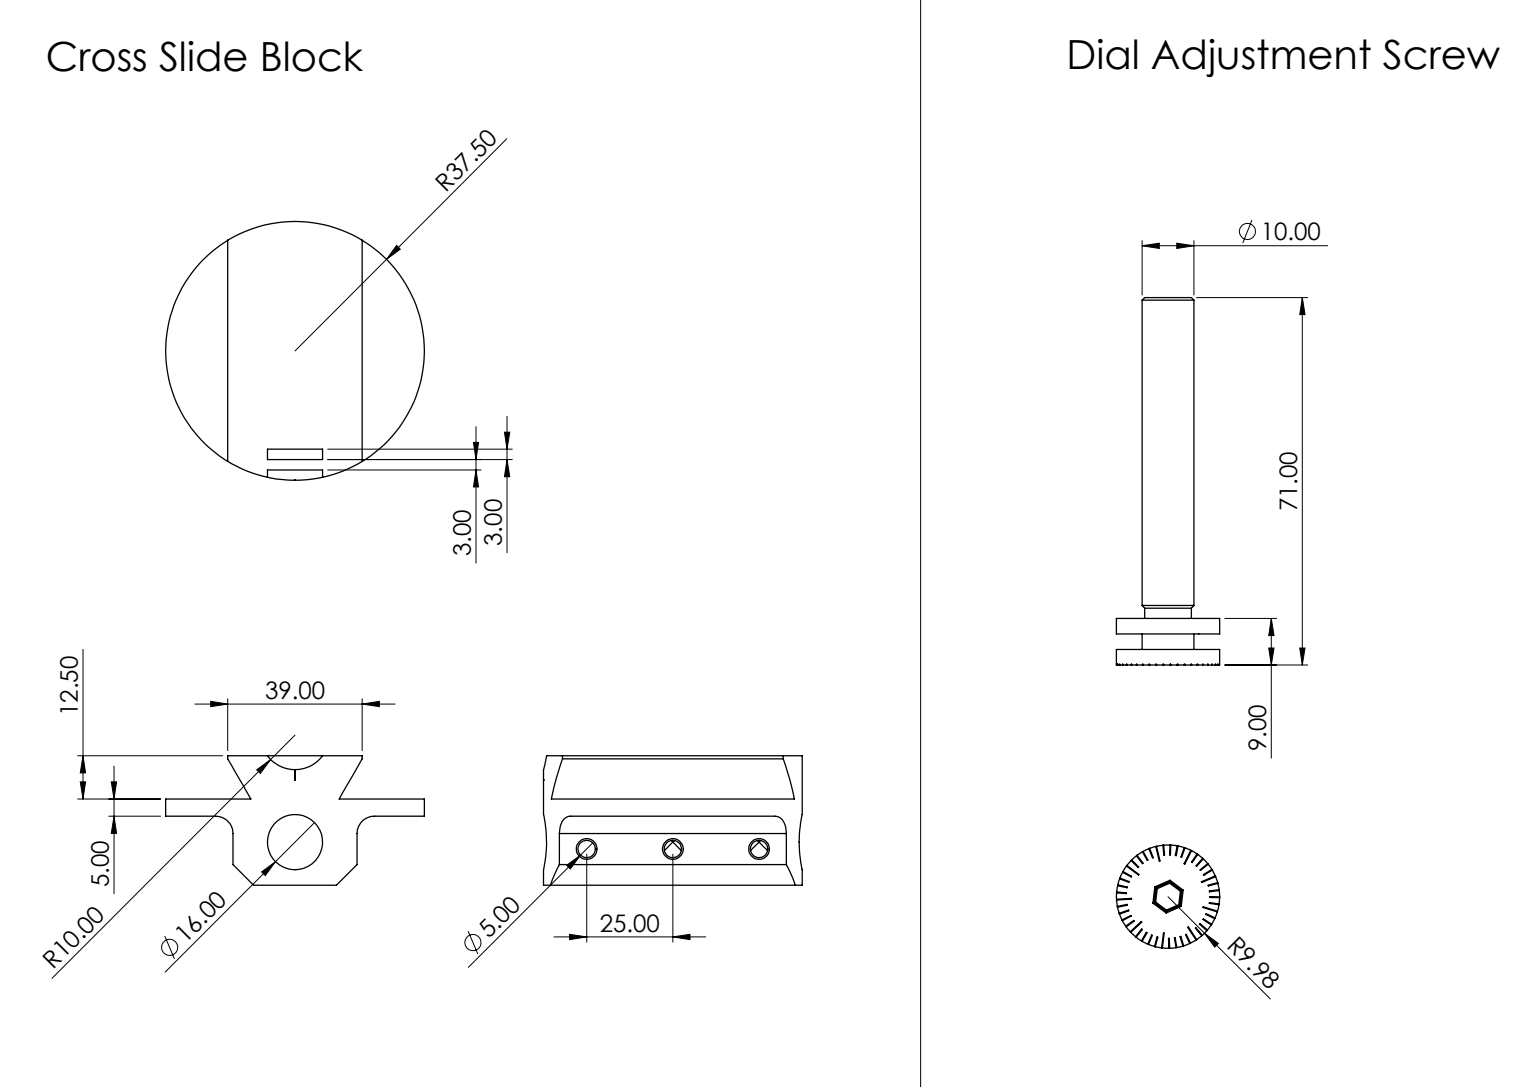
ISO-10303-21;
HEADER;
FILE_DESCRIPTION (('STEP AP214'),
    '1' );
FILE_NAME ('Cross Slide Block.step',
    '2026-10-09T18:50:44',
    ( '' ),
    ( '' ),
    'SwSTEP 2.0',
    'SolidWorks 2026',
    '' );
FILE_SCHEMA (( 'AUTOMOTIVE_DESIGN' ));
ENDSEC;

DATA;
#2=ADVANCED_FACE ( 'NONE', ( #7489 ), #472, .F. ) ;
#3=FACE_OUTER_BOUND ( 'NONE', #3774, .T. ) ;
#5=( BOUNDED_CURVE ( )  B_SPLINE_CURVE ( 3, ( #1335, #9589, #4703, #9365 ),
 .UNSPECIFIED., .F., .F. ) 
 B_SPLINE_CURVE_WITH_KNOTS ( ( 4, 4 ),
 ( 1.628044839356179940, 3.141592653589793116 ),
 .UNSPECIFIED. ) 
 CURVE ( )  GEOMETRIC_REPRESENTATION_ITEM ( )  RATIONAL_B_SPLINE_CURVE ( ( 1.000000000000000000, 0.8180365063541270576, 0.8180365063541270576, 1.000000000000000000 ) ) 
 REPRESENTATION_ITEM ( '' )  );
#9=CARTESIAN_POINT ( 'NONE',  ( -36.90121799483238618, -37.26927769664154511, 50.29562344872909563 ) ) ;
#16=EDGE_CURVE ( 'NONE', #234, #9567, #717, .T. ) ;
#23=CARTESIAN_POINT ( 'NONE',  ( 2.500300139188999182, -51.00737899243799944, -13.39525803434800011 ) ) ;
#28=CARTESIAN_POINT ( 'NONE',  ( -21.52984724227062685, -49.79067269186487721, -17.51158402248789869 ) ) ;
#37=CARTESIAN_POINT ( 'NONE',  ( -15.57469986081333424, -23.50709773848279482, 57.00223526477140013 ) ) ;
#38=EDGE_CURVE ( 'NONE', #4941, #11428, #1756, .T. ) ;
#42=CARTESIAN_POINT ( 'NONE',  ( -7.506852801849951184, -44.86566843535796778, 21.38792573514972872 ) ) ;
#48=EDGE_LOOP ( 'NONE', ( #7800, #11011, #11564, #11938, #6650, #9579, #4015 ) ) ;
#51=FACE_BOUND ( 'NONE', #14476, .T. ) ;
#53=CARTESIAN_POINT ( 'NONE',  ( -10.22150846799388191, -38.48997916076172743, -17.62493476913342150 ) ) ;
#64=VECTOR ( 'NONE', #10695, 1000.000000000000000 ) ;
#74=CARTESIAN_POINT ( 'NONE',  ( -5.499699860811000818, -46.50737899243799944, 22.50231026484399877 ) ) ;
#82=FACE_OUTER_BOUND ( 'NONE', #1702, .T. ) ;
#95=ORIENTED_EDGE ( 'NONE', *, *, #10374, .T. ) ;
#99=( BOUNDED_CURVE ( )  B_SPLINE_CURVE ( 3, ( #13212, #2486, #10670, #275 ),
 .UNSPECIFIED., .F., .T. ) 
 B_SPLINE_CURVE_WITH_KNOTS ( ( 4, 4 ),
 ( 4.712388980384689674, 6.283185307179586232 ),
 .UNSPECIFIED. ) 
 CURVE ( )  GEOMETRIC_REPRESENTATION_ITEM ( )  RATIONAL_B_SPLINE_CURVE ( ( 1.000000000000000000, 0.8047378541243649375, 0.8047378541243649375, 1.000000000000000000 ) ) 
 REPRESENTATION_ITEM ( '' )  );
#104=AXIS2_PLACEMENT_3D ( 'NONE', #5495, #8007, #12779 ) ;
#108=ORIENTED_EDGE ( 'NONE', *, *, #1414, .F. ) ;
#111=AXIS2_PLACEMENT_3D ( 'NONE', #10208, #14881, #11508 ) ;
#112=ORIENTED_EDGE ( 'NONE', *, *, #3083, .T. ) ;
#116=CARTESIAN_POINT ( 'NONE',  ( 4.650967236384746073, -37.88568168827513460, 51.12989147907354948 ) ) ;
#125=CARTESIAN_POINT ( 'NONE',  ( -7.500433020662222283, -49.00523987278725713, -5.609464624471996785 ) ) ;
#126=LINE ( 'NONE', #11658, #7291 ) ;
#128=DIRECTION ( 'NONE',  ( 0.000000000000000000, 0.000000000000000000, -1.000000000000000000 ) ) ;
#151=CARTESIAN_POINT ( 'NONE',  ( 2.500300139188999182, -51.00737899243799944, -13.39525803434800011 ) ) ;
#153=CARTESIAN_POINT ( 'NONE',  ( -28.28282149594069850, -32.00737899243799944, -17.99768973515599768 ) ) ;
#162=LINE ( 'NONE', #9710, #2630 ) ;
#163=CARTESIAN_POINT ( 'NONE',  ( -37.26807582031575805, -37.15669500878452425, 50.03818627108570638 ) ) ;
#172=ORIENTED_EDGE ( 'NONE', *, *, #3900, .F. ) ;
#174=CARTESIAN_POINT ( 'NONE',  ( -15.49969986081099904, -44.50737899243799944, -109.5506571639849938 ) ) ;
#177=EDGE_CURVE ( 'NONE', #13055, #12587, #8525, .T. ) ;
#182=CARTESIAN_POINT ( 'NONE',  ( 4.224496369445544630, -38.22985747236960918, -12.39136299437819488 ) ) ;
#187=CARTESIAN_POINT ( 'NONE',  ( 2.883830742001312508, -40.08477038827061989, 52.18712618527332125 ) ) ;
#189=CIRCLE ( 'NONE', #12147, 2.499999999999999556 ) ;
#199=EDGE_LOOP ( 'NONE', ( #11824, #6464, #11368, #3598 ) ) ;
#202=CARTESIAN_POINT ( 'NONE',  ( -7.499699860810999041, -19.50737899243799589, 51.00231026484400587 ) ) ;
#206=CARTESIAN_POINT ( 'NONE',  ( -16.55248250669792753, -52.45523696625489407, 56.99108552064786437 ) ) ;
#208=( NAMED_UNIT ( * ) SI_UNIT ( $, .STERADIAN. ) SOLID_ANGLE_UNIT ( ) );
#213=CARTESIAN_POINT ( 'NONE',  ( -15.49969986081099016, -52.50737899243799944, 27.50231026484399521 ) ) ;
#214=EDGE_CURVE ( 'NONE', #2810, #1679, #14130, .T. ) ;
#226=CARTESIAN_POINT ( 'NONE',  ( -15.49969986081098838, -17.75737899243799944, 48.00231026484399877 ) ) ;
#229=CARTESIAN_POINT ( 'NONE',  ( -7.753733168396170328, -46.50737899243799944, 47.00231026484399877 ) ) ;
#231=AXIS2_PLACEMENT_3D ( 'NONE', #5849, #3193, #3340 ) ;
#232=PLANE ( 'NONE',  #13853 ) ;
#234=VERTEX_POINT ( 'NONE', #10472 ) ;
#237=CARTESIAN_POINT ( 'NONE',  ( -15.49969986081099727, -52.50737899243799944, 2.502310264843994769 ) ) ;
#240=VECTOR ( 'NONE', #12413, 1000.000000000000000 ) ;
#243=ORIENTED_EDGE ( 'NONE', *, *, #13545, .T. ) ;
#244=ORIENTED_EDGE ( 'NONE', *, *, #12022, .T. ) ;
#253=CIRCLE ( 'NONE', #14173, 37.50000000000000000 ) ;
#260=ORIENTED_EDGE ( 'NONE', *, *, #6343, .T. ) ;
#261=CARTESIAN_POINT ( 'NONE',  ( 5.515696375138871232, -37.41693849659856141, 50.56059116161328859 ) ) ;
#272=CARTESIAN_POINT ( 'NONE',  ( -7.749729581313432369, -48.02091033734640035, -3.487279356396127739 ) ) ;
#273=CARTESIAN_POINT ( 'NONE',  ( -34.99969986081099904, -19.50737899243800300, 51.53354502093799994 ) ) ;
#275=CARTESIAN_POINT ( 'NONE',  ( -15.49969986081099727, -36.50737899243799944, 2.502310264843996546 ) ) ;
#279=CARTESIAN_POINT ( 'NONE',  ( -5.499699860811003482, -46.50737899243799944, 44.50231026484399877 ) ) ;
#281=CARTESIAN_POINT ( 'NONE',  ( -14.45170227088251202, -36.55910949265851428, -17.98655532003696678 ) ) ;
#283=EDGE_CURVE ( 'NONE', #10750, #11940, #6056, .T. ) ;
#285=DIRECTION ( 'NONE',  ( 0.000000000000000000, 0.000000000000000000, -1.000000000000000000 ) ) ;
#297=ORIENTED_EDGE ( 'NONE', *, *, #1602, .F. ) ;
#299=ORIENTED_EDGE ( 'NONE', *, *, #12335, .F. ) ;
#314=ADVANCED_FACE ( 'NONE', ( #7004, #5865, #10542, #6834 ), #10286, .F. ) ;
#318=ORIENTED_EDGE ( 'NONE', *, *, #7751, .T. ) ;
#338=CARTESIAN_POINT ( 'NONE',  ( -15.49969986081099904, -57.00737899243801365, 57.00231026484399166 ) ) ;
#344=ORIENTED_EDGE ( 'NONE', *, *, #5377, .F. ) ;
#363=CARTESIAN_POINT ( 'NONE',  ( -19.50440554761897261, -37.57692853466172522, 56.78858631758297548 ) ) ;
#376=DIRECTION ( 'NONE',  ( 0.000000000000000000, 0.000000000000000000, 1.000000000000000000 ) ) ;
#379=PLANE ( 'NONE',  #13903 ) ;
#384=DIRECTION ( 'NONE',  ( 0.000000000000000000, -1.000000000000000000, -1.224646799147350002E-16 ) ) ;
#386=CARTESIAN_POINT ( 'NONE',  ( -7.813858722443232097, -47.64803766822201680, 17.27706589258430014 ) ) ;
#387=LINE ( 'NONE', #9553, #4308 ) ;
#390=CARTESIAN_POINT ( 'NONE',  ( -7.921791253741313987, -47.08507903579843656, -17.22412991407007254 ) ) ;
#393=EDGE_CURVE ( 'NONE', #2126, #6515, #10210, .T. ) ;
#397=CARTESIAN_POINT ( 'NONE',  ( -33.53898029810832782, -41.37673382704548430, -13.37373704449904999 ) ) ;
#399=ORIENTED_EDGE ( 'NONE', *, *, #9618, .F. ) ;
#410=SHAPE_REPRESENTATION ( 'Cross Slide Block', ( #6789 ), #14627 ) ;
#411=DIRECTION ( 'NONE',  ( 0.000000000000000000, -1.000000000000000000, -1.224646799147350002E-16 ) ) ;
#424=CARTESIAN_POINT ( 'NONE',  ( -7.499751500627866996, -49.00722532478560822, -5.529656340655102476 ) ) ;
#427=CARTESIAN_POINT ( 'NONE',  ( 2.500300139188998738, -46.50737899243799944, 22.00231026484399877 ) ) ;
#435=ADVANCED_FACE ( 'NONE', ( #3259 ), #11815, .F. ) ;
#437=CARTESIAN_POINT ( 'NONE',  ( -9.503465417293824657, -21.51087798686868169, 56.51956357228300476 ) ) ;
#455=AXIS2_PLACEMENT_3D ( 'NONE', #5725, #6934, #3584 ) ;
#458=ADVANCED_FACE ( 'NONE', ( #3557 ), #9287, .T. ) ;
#459=CARTESIAN_POINT ( 'NONE',  ( -7.879287384819388507, -47.08648443922106708, 17.06717620651851064 ) ) ;
#461=DIRECTION ( 'NONE',  ( -1.000000000000000000, 1.291538348938060198E-32, -1.054621095516909827E-16 ) ) ;
#463=DIRECTION ( 'NONE',  ( 0.000000000000000000, 0.000000000000000000, 1.000000000000000000 ) ) ;
#468=CARTESIAN_POINT ( 'NONE',  ( -37.32932784798677517, -37.10979894228395182, -10.99641364132881094 ) ) ;
#472=CYLINDRICAL_SURFACE ( 'NONE', #13911, 10.00000000000000000 ) ;
#477=CYLINDRICAL_SURFACE ( 'NONE', #7239, 2.500000000000002220 ) ;
#483=CARTESIAN_POINT ( 'NONE',  ( -7.506367692296740834, -44.17806943360024974, 45.42009090809814609 ) ) ;
#486=CARTESIAN_POINT ( 'NONE',  ( -1.425463962227843995, -54.93314309385483796, 54.32987364559348009 ) ) ;
#496=( BOUNDED_CURVE ( )  B_SPLINE_CURVE ( 3, ( #7778, #12464, #6703, #906 ),
 .UNSPECIFIED., .F., .F. ) 
 B_SPLINE_CURVE_WITH_KNOTS ( ( 4, 4 ),
 ( 1.570796326794895004, 3.141592653589793116 ),
 .UNSPECIFIED. ) 
 CURVE ( )  GEOMETRIC_REPRESENTATION_ITEM ( )  RATIONAL_B_SPLINE_CURVE ( ( 1.000000000000000000, 0.8047378541243646044, 0.8047378541243646044, 1.000000000000000000 ) ) 
 REPRESENTATION_ITEM ( '' )  );
#504=CARTESIAN_POINT ( 'NONE',  ( -21.84916367058906772, -49.38105347906694931, 56.46124168193669135 ) ) ;
#515=EDGE_CURVE ( 'NONE', #12112, #5496, #126, .T. ) ;
#518=ORIENTED_EDGE ( 'NONE', *, *, #13012, .T. ) ;
#521=CARTESIAN_POINT ( 'NONE',  ( -7.838590061662593200, -46.81644859005926662, 21.98773677246508740 ) ) ;
#542=PRODUCT_DEFINITION_SHAPE ( 'NONE', 'NONE',  #10680 ) ;
#546=CARTESIAN_POINT ( 'NONE',  ( -5.499699860811000818, -46.50737899243799944, 22.50231026484399877 ) ) ;
#548=FACE_OUTER_BOUND ( 'NONE', #4580, .T. ) ;
#569=VERTEX_POINT ( 'NONE', #273 ) ;
#570=CARTESIAN_POINT ( 'NONE',  ( -15.49969986081099371, -26.50737899243800300, 56.85231026484400019 ) ) ;
#573=CARTESIAN_POINT ( 'NONE',  ( -5.499699860810998153, -46.50737899243799944, -2.497689735156003010 ) ) ;
#576=CARTESIAN_POINT ( 'NONE',  ( -18.33272512729327985, -51.99348705970457729, 56.89592189784066534 ) ) ;
#577=ORIENTED_EDGE ( 'NONE', *, *, #2278, .F. ) ;
#578=CARTESIAN_POINT ( 'NONE',  ( -14.97634376076197427, -36.52016005446672864, 56.99957717010889269 ) ) ;
#589=DIRECTION ( 'NONE',  ( -3.839882694219489529E-17, 1.000000000000000000, 0.000000000000000000 ) ) ;
#603=CARTESIAN_POINT ( 'NONE',  ( 2.500300139188996962, -46.50737899243799944, 41.50231026484399166 ) ) ;
#608=VECTOR ( 'NONE', #7086, 1000.000000000000000 ) ;
#610=CARTESIAN_POINT ( 'NONE',  ( -35.12686845230359722, -38.31628777931871355, -12.45116519455210202 ) ) ;
#623=CARTESIAN_POINT ( 'NONE',  ( -7.500891366873055688, -44.35589769198639942, 43.22203397690024218 ) ) ;
#624=ORIENTED_EDGE ( 'NONE', *, *, #10374, .F. ) ;
#632=DIRECTION ( 'NONE',  ( 0.000000000000000000, 0.000000000000000000, -1.000000000000000000 ) ) ;
#648=EDGE_LOOP ( 'NONE', ( #4869, #13209, #1415, #10166, #10438, #12905, #14791, #3642, #7670 ) ) ;
#649=CARTESIAN_POINT ( 'NONE',  ( -13.41733751443047318, -36.76536173621014569, 56.94798727393903448 ) ) ;
#654=AXIS2_PLACEMENT_3D ( 'NONE', #10348, #4542, #5827 ) ;
#658=FACE_OUTER_BOUND ( 'NONE', #3242, .T. ) ;
#661=ORIENTED_EDGE ( 'NONE', *, *, #914, .T. ) ;
#677=CARTESIAN_POINT ( 'NONE',  ( -7.557949836157023427, -45.46309933671603432, -3.215436967628607867 ) ) ;
#681=FACE_OUTER_BOUND ( 'NONE', #12815, .T. ) ;
#684=EDGE_CURVE ( 'NONE', #5678, #1019, #2058, .T. ) ;
#687=CARTESIAN_POINT ( 'NONE',  ( -11.90127153857800302, -52.50737899243802786, 27.50231026484402719 ) ) ;
#697=CARTESIAN_POINT ( 'NONE',  ( -7.499699860810999041, -44.50737899243799944, 43.00231026484400587 ) ) ;
#698=ORIENTED_EDGE ( 'NONE', *, *, #7230, .T. ) ;
#702=CARTESIAN_POINT ( 'NONE',  ( -7.661871090851159138, -46.13481490855701139, -7.997691309909533253 ) ) ;
#716=CARTESIAN_POINT ( 'NONE',  ( -34.99969986081099904, -19.50737899243800300, -12.52892449124999885 ) ) ;
#717=CIRCLE ( 'NONE', #11214, 2.999999999999999112 ) ;
#720=LINE ( 'NONE', #573, #13845 ) ;
#724=CARTESIAN_POINT ( 'NONE',  ( -19.51359857101742534, -51.44753102027924285, 56.78947505621691505 ) ) ;
#728=DIRECTION ( 'NONE',  ( -1.000000000000000000, 1.291538348938060198E-32, -1.054621095516909827E-16 ) ) ;
#733=CARTESIAN_POINT ( 'NONE',  ( -20.18599136182623965, -36.50737899243796392, 11.50231026484396146 ) ) ;
#734=DIRECTION ( 'NONE',  ( 1.000000000000000000, -1.291538348938060198E-32, 1.054621095516909827E-16 ) ) ;
#755=ORIENTED_EDGE ( 'NONE', *, *, #9574, .T. ) ;
#759=ADVANCED_FACE ( 'NONE', ( #4504 ), #3350, .F. ) ;
#761=CARTESIAN_POINT ( 'NONE',  ( -33.81822260959295789, -40.24903322724137666, -13.21898423093114161 ) ) ;
#762=ORIENTED_EDGE ( 'NONE', *, *, #283, .F. ) ;
#765=CARTESIAN_POINT ( 'NONE',  ( -12.67205704361948193, -51.99558085209910985, 56.89633976960556083 ) ) ;
#767=CARTESIAN_POINT ( 'NONE',  ( -15.49969986081099904, -37.00737899243799944, 19.50231026484400232 ) ) ;
#768=CARTESIAN_POINT ( 'NONE',  ( -15.49969986081100082, -19.50737899243800300, 19.50231026484399877 ) ) ;
#777=VERTEX_POINT ( 'NONE', #12850 ) ;
#780=CARTESIAN_POINT ( 'NONE',  ( -7.794854316102236780, -46.66267709929380914, 17.00231091965724062 ) ) ;
#790=AXIS2_PLACEMENT_3D ( 'NONE', #1874, #14724, #12284 ) ;
#795=CARTESIAN_POINT ( 'NONE',  ( -15.49969986081099727, -57.00737899243800655, 2.502310264843997878 ) ) ;
#798=ORIENTED_EDGE ( 'NONE', *, *, #9757, .T. ) ;
#802=CARTESIAN_POINT ( 'NONE',  ( 2.551851194784686250, -41.28719780953740326, 52.37162401788530985 ) ) ;
#804=CARTESIAN_POINT ( 'NONE',  ( -20.06287389993751447, -22.40558212242008196, 56.72366690358678909 ) ) ;
#809=ADVANCED_FACE ( 'NONE', ( #11215 ), #3022, .F. ) ;
#815=DIRECTION ( 'NONE',  ( 1.000000000000000000, -1.291538348938060198E-32, 1.054621095516909827E-16 ) ) ;
#818=VERTEX_POINT ( 'NONE', #7533 ) ;
#823=CARTESIAN_POINT ( 'NONE',  ( -19.05470409992778258, -37.32136930023363419, -17.83198480484461967 ) ) ;
#835=CARTESIAN_POINT ( 'NONE',  ( 2.500300139188999626, -46.50737899243799944, 42.00231026484399166 ) ) ;
#842=STYLED_ITEM ( 'NONE', ( #11744 ), #12764 ) ;
#846=DIRECTION ( 'NONE',  ( 0.000000000000000000, -1.000000000000000000, -1.224646799147350002E-16 ) ) ;
#851=CARTESIAN_POINT ( 'NONE',  ( -5.499699860811000818, -46.50737899243799944, 17.00231026484399877 ) ) ;
#855=VERTEX_POINT ( 'NONE', #11283 ) ;
#861=DIRECTION ( 'NONE',  ( -1.000000000000000000, 1.291538348938060198E-32, -1.054621095516909827E-16 ) ) ;
#863=DIRECTION ( 'NONE',  ( 0.000000000000000000, 0.000000000000000000, 1.000000000000000000 ) ) ;
#871=CARTESIAN_POINT ( 'NONE',  ( -23.49969986081100259, -44.50737899243799944, 56.13904046828872652 ) ) ;
#885=CARTESIAN_POINT ( 'NONE',  ( -7.754930580632606762, -46.50765881518451295, 22.00225574842814424 ) ) ;
#886=CYLINDRICAL_SURFACE ( 'NONE', #3992, 2.500000000000002220 ) ;
#888=ORIENTED_EDGE ( 'NONE', *, *, #9875, .T. ) ;
#894=LINE ( 'NONE', #10136, #2389 ) ;
#900=DIRECTION ( 'NONE',  ( -1.000000000000000000, 1.291538348938060198E-32, -1.054621095516909827E-16 ) ) ;
#906=CARTESIAN_POINT ( 'NONE',  ( -15.49969986081099904, -52.50737899243800655, -13.49768973515600656 ) ) ;
#911=CARTESIAN_POINT ( 'NONE',  ( -7.502222146387037327, -44.75835849886513529, 46.29929020896280178 ) ) ;
#914=EDGE_CURVE ( 'NONE', #1019, #12480, #14071, .T. ) ;
#919=DIRECTION ( 'NONE',  ( 0.000000000000000000, 1.000000000000000000, 1.224646799147350002E-16 ) ) ;
#920=CARTESIAN_POINT ( 'NONE',  ( -7.949560932996365459, -47.15762953262321844, 42.08283266251152810 ) ) ;
#935=DIRECTION ( 'NONE',  ( 0.000000000000000000, 1.224646799147350002E-16, -1.000000000000000000 ) ) ;
#941=LINE ( 'NONE', #3154, #7567 ) ;
#944=CARTESIAN_POINT ( 'NONE',  ( -7.813858722443190352, -47.64803766822263498, -7.722934107415373006 ) ) ;
#946=CYLINDRICAL_SURFACE ( 'NONE', #13032, 8.000000000000000000 ) ;
#954=CARTESIAN_POINT ( 'NONE',  ( 2.704135510968567857, -40.58388572175281439, 52.28758934844383077 ) ) ;
#957=B_SPLINE_CURVE_WITH_KNOTS ( 'NONE', 3,
 ( #7231, #11916, #1439, #3884, #6166, #3805 ),
 .UNSPECIFIED., .F., .F.,
 ( 4, 2, 4 ),
 ( 0.000000000000000000, 0.1440237844040733739, 0.2880475688081467478 ),
 .UNSPECIFIED. ) ;
#960=EDGE_CURVE ( 'NONE', #7202, #3278, #2137, .T. ) ;
#961=CARTESIAN_POINT ( 'NONE',  ( -7.557932192427426088, -45.46324534594638322, 21.78464076912158376 ) ) ;
#978=CARTESIAN_POINT ( 'NONE',  ( -7.611722567307242393, -48.62974432432149285, 20.82618560148544518 ) ) ;
#992=CARTESIAN_POINT ( 'NONE',  ( -8.703303756061691487, -48.73563719200068078, 56.38158717348355253 ) ) ;
#998=CYLINDRICAL_SURFACE ( 'NONE', #3816, 8.000000000000000000 ) ;
#1000=CARTESIAN_POINT ( 'NONE',  ( -5.499699860811003482, -46.50737899243799944, 47.50231026484399877 ) ) ;
#1001=ORIENTED_EDGE ( 'NONE', *, *, #9257, .F. ) ;
#1007=ORIENTED_EDGE ( 'NONE', *, *, #2915, .T. ) ;
#1013=EDGE_CURVE ( 'NONE', #12480, #7811, #6818, .T. ) ;
#1015=CARTESIAN_POINT ( 'NONE',  ( -23.49969986081100259, -44.50737899243799944, -17.13441993860073254 ) ) ;
#1016=ADVANCED_FACE ( 'NONE', ( #14955 ), #11362, .F. ) ;
#1019=VERTEX_POINT ( 'NONE', #12667 ) ;
#1026=ORIENTED_EDGE ( 'NONE', *, *, #9723, .F. ) ;
#1028=CARTESIAN_POINT ( 'NONE',  ( -23.49969986081099904, -19.50737899243800300, 56.13904046828879757 ) ) ;
#1032=VECTOR ( 'NONE', #384, 1000.000000000000000 ) ;
#1033=AXIS2_PLACEMENT_3D ( 'NONE', #10244, #1067, #9318 ) ;
#1036=CARTESIAN_POINT ( 'NONE',  ( -23.49969986081100615, -39.82108749142274462, 24.18860176585925359 ) ) ;
#1045=CARTESIAN_POINT ( 'NONE',  ( -33.49969986081099904, -37.00737899243799944, 52.39987856403599409 ) ) ;
#1050=DIRECTION ( 'NONE',  ( 0.000000000000000000, 0.000000000000000000, -1.000000000000000000 ) ) ;
#1055=DIRECTION ( 'NONE',  ( 1.000000000000000000, -1.291538348938060198E-32, 1.054621095516909827E-16 ) ) ;
#1056=ORIENTED_EDGE ( 'NONE', *, *, #12207, .F. ) ;
#1058=DIRECTION ( 'NONE',  ( 0.000000000000000000, -1.000000000000000000, -1.224646799147350002E-16 ) ) ;
#1067=DIRECTION ( 'NONE',  ( -1.000000000000000000, 1.291538348938060198E-32, -1.054621095516909827E-16 ) ) ;
#1071=( BOUNDED_CURVE ( )  B_SPLINE_CURVE ( 3, ( #5218, #486, #9882, #9806 ),
 .UNSPECIFIED., .F., .T. ) 
 B_SPLINE_CURVE_WITH_KNOTS ( ( 4, 4 ),
 ( 5.038118467679318258, 5.213043692789277372 ),
 .UNSPECIFIED. ) 
 CURVE ( )  GEOMETRIC_REPRESENTATION_ITEM ( )  RATIONAL_B_SPLINE_CURVE ( ( 1.000000000000000000, 0.9974517222217438306, 0.9974517222217438306, 1.000000000000000000 ) ) 
 REPRESENTATION_ITEM ( '' )  );
#1081=EDGE_LOOP ( 'NONE', ( #9027, #14553, #6370, #10972 ) ) ;
#1084=DIRECTION ( 'NONE',  ( 0.000000000000000000, 0.000000000000000000, 1.000000000000000000 ) ) ;
#1099=CARTESIAN_POINT ( 'NONE',  ( -7.768926039458098565, -39.58069824233446354, 24.42899101494754888 ) ) ;
#1102=DIRECTION ( 'NONE',  ( 3.632077277826439854E-16, -1.000000000000000000, 0.000000000000000000 ) ) ;
#1104=CARTESIAN_POINT ( 'NONE',  ( -15.49969986081099016, -36.50737899243799944, 27.50231026484399521 ) ) ;
#1108=CARTESIAN_POINT ( 'NONE',  ( -7.595066331666822990, -45.75350114379759958, 42.11098092323300790 ) ) ;
#1113=CARTESIAN_POINT ( 'NONE',  ( -19.51357682882387934, -37.56763829276790290, -17.78480384862011832 ) ) ;
#1124=ORIENTED_EDGE ( 'NONE', *, *, #3060, .F. ) ;
#1130=CARTESIAN_POINT ( 'NONE',  ( -7.529934156977152959, -45.22371508067976720, 46.65625893024207471 ) ) ;
#1132=CARTESIAN_POINT ( 'NONE',  ( -7.512805849530849400, -44.04964101872670312, 19.04457229113268113 ) ) ;
#1137=CARTESIAN_POINT ( 'NONE',  ( -7.845610686729125760, -46.84038939242768151, 46.98533734250990790 ) ) ;
#1141=ADVANCED_FACE ( 'NONE', ( #8364 ), #8443, .T. ) ;
#1156=CARTESIAN_POINT ( 'NONE',  ( -7.512805849530849400, -44.04964101872670312, -5.955427708867301106 ) ) ;
#1161=CARTESIAN_POINT ( 'NONE',  ( -5.499699860811000818, -46.50737899243799944, 19.50231026484399877 ) ) ;
#1163=DIRECTION ( 'NONE',  ( 0.000000000000000000, 0.000000000000000000, -1.000000000000000000 ) ) ;
#1166=CARTESIAN_POINT ( 'NONE',  ( 3.909245658297777037, -38.51142663664874277, -12.58558199649565168 ) ) ;
#1182=CARTESIAN_POINT ( 'NONE',  ( 2.500300139188998738, -46.50737899243799944, 22.50231026484399877 ) ) ;
#1185=ORIENTED_EDGE ( 'NONE', *, *, #4087, .T. ) ;
#1194=SURFACE_STYLE_FILL_AREA ( #5924 ) ;
#1203=ORIENTED_EDGE ( 'NONE', *, *, #14579, .T. ) ;
#1206=CARTESIAN_POINT ( 'NONE',  ( -15.49969986081099194, -27.00737899243800300, 11.50231026484399877 ) ) ;
#1208=LINE ( 'NONE', #3064, #4623 ) ;
#1210=CARTESIAN_POINT ( 'NONE',  ( -7.502358996163085436, -44.29392756818862154, -6.675385003928089311 ) ) ;
#1221=CARTESIAN_POINT ( 'NONE',  ( -33.49969986081099904, -42.00737899243800655, 52.39987856403599409 ) ) ;
#1223=CARTESIAN_POINT ( 'NONE',  ( -35.26908782159542000, -38.19079675818825592, 51.36802084380344979 ) ) ;
#1229=VERTEX_POINT ( 'NONE', #6489 ) ;
#1237=SHAPE_REPRESENTATION_RELATIONSHIP ( 'NONE' , 'NONE' ,  #410, #6261 ) ;
#1242=CARTESIAN_POINT ( 'NONE',  ( 7.500300139189000070, -37.00737899243799944, -10.11609617439569675 ) ) ;
#1255=CARTESIAN_POINT ( 'NONE',  ( -7.553613233656758297, -48.84439576093704716, -4.598074977179023470 ) ) ;
#1260=VERTEX_POINT ( 'NONE', #10017 ) ;
#1263=CARTESIAN_POINT ( 'NONE',  ( -19.73154169590003093, -37.71326103272679120, 56.76340952534463469 ) ) ;
#1265=( NAMED_UNIT ( * ) PLANE_ANGLE_UNIT ( ) SI_UNIT ( $, .RADIAN. ) );
#1267=CIRCLE ( 'NONE', #2254, 37.50000000000000000 ) ;
#1293=EDGE_CURVE ( 'NONE', #2996, #2185, #9966, .T. ) ;
#1297=CARTESIAN_POINT ( 'NONE',  ( -15.49969986081099904, -44.50737899243799944, -109.5506571639849938 ) ) ;
#1311=ORIENTED_EDGE ( 'NONE', *, *, #9300, .T. ) ;
#1335=CARTESIAN_POINT ( 'NONE',  ( -7.512805849530849400, -44.04964101872670312, -5.955427708867301106 ) ) ;
#1339=CARTESIAN_POINT ( 'NONE',  ( -7.508350897672356972, -44.16519039693573490, 20.39701027657645227 ) ) ;
#1348=CARTESIAN_POINT ( 'NONE',  ( -15.49969986081099904, -52.50737899243799944, 57.00231026484399166 ) ) ;
#1356=VERTEX_POINT ( 'NONE', #3594 ) ;
#1358=DIRECTION ( 'NONE',  ( 0.000000000000000000, 0.000000000000000000, -1.000000000000000000 ) ) ;
#1362=ORIENTED_EDGE ( 'NONE', *, *, #12175, .T. ) ;
#1385=VERTEX_POINT ( 'NONE', #14075 ) ;
#1389=DIRECTION ( 'NONE',  ( 0.000000000000000000, -1.000000000000000000, -1.224646799147350002E-16 ) ) ;
#1395=CARTESIAN_POINT ( 'NONE',  ( 4.180649471280372786, -38.26834254388227663, -12.41843850008141992 ) ) ;
#1412=CARTESIAN_POINT ( 'NONE',  ( -7.503901077028577227, -48.99487332462116740, -5.755859045742772295 ) ) ;
#1414=EDGE_CURVE ( 'NONE', #855, #11014, #5593, .T. ) ;
#1415=ORIENTED_EDGE ( 'NONE', *, *, #4203, .T. ) ;
#1417=EDGE_CURVE ( 'NONE', #3424, #6799, #8006, .T. ) ;
#1418=AXIS2_PLACEMENT_3D ( 'NONE', #10149, #14679, #8781 ) ;
#1427=FILL_AREA_STYLE_COLOUR ( '', #13311 ) ;
#1431=CARTESIAN_POINT ( 'NONE',  ( -7.499699860810999041, -19.50737899243799589, 56.13904046828879757 ) ) ;
#1432=AXIS2_PLACEMENT_3D ( 'NONE', #9239, #3665, #8319 ) ;
#1434=CARTESIAN_POINT ( 'NONE',  ( -23.49969986081099194, -49.19367049345326137, 24.18860176585926425 ) ) ;
#1438=ORIENTED_EDGE ( 'NONE', *, *, #11015, .F. ) ;
#1439=CARTESIAN_POINT ( 'NONE',  ( -7.508318444979633632, -44.14098664639713832, 18.67373629545663150 ) ) ;
#1442=CARTESIAN_POINT ( 'NONE',  ( -23.49969986081099904, -44.50737899243799944, 19.50231026484399877 ) ) ;
#1444=CARTESIAN_POINT ( 'NONE',  ( -15.49969986081099194, -57.00737899243800655, 11.50231026484399521 ) ) ;
#1452=CARTESIAN_POINT ( 'NONE',  ( -8.313210069164949090, -48.06114224692424841, -17.30321196480585400 ) ) ;
#1456=CARTESIAN_POINT ( 'NONE',  ( -7.508347634011948379, -44.16528234937342035, -4.602730171981503915 ) ) ;
#1458=ORIENTED_EDGE ( 'NONE', *, *, #8209, .T. ) ;
#1464=EDGE_LOOP ( 'NONE', ( #6842, #9273, #8453, #1056 ) ) ;
#1465=CARTESIAN_POINT ( 'NONE',  ( -7.754930580632606762, -46.50765881518451295, 22.00225574842814424 ) ) ;
#1480=CARTESIAN_POINT ( 'NONE',  ( 6.906785209640905698, -37.00737899243799944, 49.58160724549794196 ) ) ;
#1490=CARTESIAN_POINT ( 'NONE',  ( -7.705418609684434372, -48.24386234041418220, -3.676323684936692260 ) ) ;
#1493=CARTESIAN_POINT ( 'NONE',  ( -7.501944906337848273, -44.50613385756380325, -4.001965388595783324 ) ) ;
#1494=CARTESIAN_POINT ( 'NONE',  ( -34.99969986081099904, -20.37340439622244048, 51.53354502093799994 ) ) ;
#1502=DIRECTION ( 'NONE',  ( -1.000000000000000000, 1.291538348938060198E-32, -1.054621095516909827E-16 ) ) ;
#1505=CARTESIAN_POINT ( 'NONE',  ( -11.14685911689329245, -22.51056837233514329, 56.74883337938142347 ) ) ;
#1507=CARTESIAN_POINT ( 'NONE',  ( -20.18599136182622544, -52.50737899243804918, 27.50231026484403429 ) ) ;
#1516=VERTEX_POINT ( 'NONE', #5194 ) ;
#1520=CARTESIAN_POINT ( 'NONE',  ( -15.49969986081099904, -36.50737899243799944, -13.49768973515600479 ) ) ;
#1522=CARTESIAN_POINT ( 'NONE',  ( -7.690624001724057912, -48.30857337213000591, 17.76824091595882393 ) ) ;
#1523=AXIS2_PLACEMENT_3D ( 'NONE', #11146, #10059, #8918 ) ;
#1528=VERTEX_POINT ( 'NONE', #7408 ) ;
#1537=EDGE_CURVE ( 'NONE', #2093, #11647, #5320, .T. ) ;
#1548=AXIS2_PLACEMENT_3D ( 'NONE', #12898, #7977, #5837 ) ;
#1559=DIRECTION ( 'NONE',  ( 0.000000000000000000, 0.000000000000000000, 1.000000000000000000 ) ) ;
#1566=DIRECTION ( 'NONE',  ( 0.000000000000000000, 1.850371707708594316E-16, -1.000000000000000000 ) ) ;
#1575=CARTESIAN_POINT ( 'NONE',  ( 2.500300139188999626, -46.50737899243799944, 17.00231026484399877 ) ) ;
#1581=FACE_OUTER_BOUND ( 'NONE', #12812, .T. ) ;
#1585=EDGE_CURVE ( 'NONE', #2658, #9374, #4852, .T. ) ;
#1587=ORIENTED_EDGE ( 'NONE', *, *, #9618, .T. ) ;
#1599=CARTESIAN_POINT ( 'NONE',  ( -33.81844200665902633, -40.24211141608020625, 52.22352481299739679 ) ) ;
#1602=EDGE_CURVE ( 'NONE', #5522, #11803, #496, .T. ) ;
#1605=CARTESIAN_POINT ( 'NONE',  ( -38.49969986081099904, -37.00737899243799944, -10.11609617439569675 ) ) ;
#1615=B_SPLINE_CURVE_WITH_KNOTS ( 'NONE', 3,
 ( #1242, #6957, #4615, #9352, #3461, #8428, #8271, #2470, #3541, #7116, #2399, #14175, #12811, #11799, #5978, #7268, #182, #11957, #1395, #1166, #10650, #10502, #4694, #14023, #8196, #4846, #7040, #10577, #4769, #4921, #9427, #3693, #13040, #7196, #11874, #6047 ),
 .UNSPECIFIED., .F., .F.,
 ( 4, 2, 1, 1, 1, 2, 2, 2, 1, 1, 1, 2, 2, 2, 2, 2, 2, 2, 2, 2, 4 ),
 ( 0.000000000000000000, 0.1249999999999999722, 0.1875000000000001110, 0.2187500000000004996, 0.2343750000000006661, 0.2421875000000008049, 0.2500000000000009437, 0.3749999999999957256, 0.4374999999999933387, 0.4687499999999920064, 0.4843749999999903966, 0.4921874999999891198, 0.4999999999999878431, 0.6249999999999860112, 0.6874999999999842348, 0.7187499999999843459, 0.7499999999999844569, 0.8124999999999865663, 0.8437499999999887867, 0.8749999999999910072, 1.000000000000000000 ),
 .UNSPECIFIED. ) ;
#1620=CARTESIAN_POINT ( 'NONE',  ( -15.57469986081099478, -26.50737899243800300, 56.85231026484400019 ) ) ;
#1621=EDGE_LOOP ( 'NONE', ( #3160, #7243 ) ) ;
#1633=AXIS2_PLACEMENT_3D ( 'NONE', #6667, #12733, #10192 ) ;
#1643=CARTESIAN_POINT ( 'NONE',  ( -21.51730450772242875, -49.78533579282670729, 56.51672281561283029 ) ) ;
#1651=CARTESIAN_POINT ( 'NONE',  ( -11.44877351069547444, -22.65069971201824828, 56.78273114525553922 ) ) ;
#1658=DIRECTION ( 'NONE',  ( -1.000000000000000000, 1.291538348938060198E-32, -1.054621095516909827E-16 ) ) ;
#1669=DIRECTION ( 'NONE',  ( -1.000000000000000000, -3.632077277826439854E-16, 0.000000000000000000 ) ) ;
#1678=CARTESIAN_POINT ( 'NONE',  ( -34.09967183693625969, -39.60750234067455722, -13.06022564672880470 ) ) ;
#1679=VERTEX_POINT ( 'NONE', #5715 ) ;
#1680=ADVANCED_FACE ( 'NONE', ( #14059 ), #10534, .F. ) ;
#1693=CARTESIAN_POINT ( 'NONE',  ( -7.514648799889656061, -44.01807676418170701, 44.76925787528261225 ) ) ;
#1698=CARTESIAN_POINT ( 'NONE',  ( -7.494881439401115841, -44.62162220065265217, -7.150567461381952761 ) ) ;
#1702=EDGE_LOOP ( 'NONE', ( #14521, #4716, #7340, #8875, #13707, #9134, #14958, #5986, #6909, #10932 ) ) ;
#1735=VERTEX_POINT ( 'NONE', #9231 ) ;
#1740=CARTESIAN_POINT ( 'NONE',  ( -7.567013331128944031, -48.78395362562287829, 18.42951909465858407 ) ) ;
#1741=B_SPLINE_CURVE_WITH_KNOTS ( 'NONE', 3,
 ( #1015, #2238, #2320, #9117, #13795, #14020, #10499, #11419, #6886, #15010, #11570, #3313, #28, #7887, #10344, #9270, #15086, #10268, #14863, #4537, #9187, #2092, #8115, #14935, #4691, #13867 ),
 .UNSPECIFIED., .F., .F.,
 ( 4, 2, 2, 2, 2, 2, 2, 2, 2, 2, 2, 2, 4 ),
 ( 0.02522174898566975285, 0.02600993856294867707, 0.02679812814022759782, 0.02837450729478542544, 0.02916269687206434619, 0.02995088644934326694, 0.03152726560390109456, 0.03231545518118000143, 0.03310364475845890830, 0.03389183433573780824, 0.03468002391301671511, 0.03625640306757453579, 0.03783278222213234954 ),
 .UNSPECIFIED. ) ;
#1747=VECTOR ( 'NONE', #6276, 1000.000000000000000 ) ;
#1751=CARTESIAN_POINT ( 'NONE',  ( 2.500300139188999182, -46.50737899243799944, -5.497689735156002122 ) ) ;
#1756=LINE ( 'NONE', #13252, #4629 ) ;
#1763=FACE_OUTER_BOUND ( 'NONE', #4849, .T. ) ;
#1779=ADVANCED_FACE ( 'NONE', ( #1581 ), #12073, .F. ) ;
#1787=EDGE_CURVE ( 'NONE', #12721, #8099, #189, .T. ) ;
#1788=AXIS2_PLACEMENT_3D ( 'NONE', #11706, #10637, #11860 ) ;
#1791=ORIENTED_EDGE ( 'NONE', *, *, #14783, .F. ) ;
#1797=CARTESIAN_POINT ( 'NONE',  ( -19.05417371652952951, -51.69327491641966787, 56.83659220636065612 ) ) ;
#1798=EDGE_CURVE ( 'NONE', #12241, #7870, #8495, .T. ) ;
#1801=CARTESIAN_POINT ( 'NONE',  ( -7.886584594865190034, -46.96511696614950182, -7.955427708867500058 ) ) ;
#1804=AXIS2_PLACEMENT_3D ( 'NONE', #11529, #1055, #10988 ) ;
#1817=DIRECTION ( 'NONE',  ( 3.632077277826439854E-16, -1.000000000000000000, 0.000000000000000000 ) ) ;
#1831=CARTESIAN_POINT ( 'NONE',  ( -35.65036695804911915, -37.88568168826260063, -12.12527094935855843 ) ) ;
#1836=B_SPLINE_CURVE_WITH_KNOTS ( 'NONE', 3,
 ( #9857, #459, #2890, #2744, #13164, #7324, #386, #12007, #9922, #3967, #8630, #14378, #5117, #8551, #14524, #1522, #7475, #12150, #2964, #8699, #7622, #13384, #1740, #10859, #5044, #3894, #13238, #7402, #6395, #12083, #11078, #14671, #6768, #7996, #2049, #10068, #3116, #978, #10226, #13679, #14820, #3040, #5633, #4191, #14750, #11233, #3195, #7839, #12531 ),
 .UNSPECIFIED., .F., .F.,
 ( 4, 2, 2, 1, 1, 2, 2, 2, 2, 1, 1, 2, 2, 2, 2, 2, 1, 2, 2, 2, 2, 2, 1, 1, 2, 2, 2, 4 ),
 ( 0.000000000000000000, 0.06249999999999369948, 0.09374999999998918920, 0.1093749999999871908, 0.1171874999999874128, 0.1210937499999866634, 0.1249999999999859279, 0.1874999999999953648, 0.2187500000000005274, 0.2343750000000031086, 0.2421875000000043299, 0.2460937500000049682, 0.2500000000000056066, 0.3750000000000073830, 0.4375000000000082712, 0.4687500000000087708, 0.4843750000000079936, 0.4921875000000084377, 0.5000000000000088818, 0.6250000000000403011, 0.6875000000000554001, 0.7187500000000633937, 0.7343750000000669464, 0.7421875000000682787, 0.7460937500000681677, 0.7500000000000679456, 0.8750000000000339728, 1.000000000000000000 ),
 .UNSPECIFIED. ) ;
#1838=CARTESIAN_POINT ( 'NONE',  ( -8.308948803761788682, -48.01658430907413333, 42.50291890924265914 ) ) ;
#1840=CARTESIAN_POINT ( 'NONE',  ( -5.499699860810997265, -46.50737899243799944, -2.997689735156003010 ) ) ;
#1843=DIRECTION ( 'NONE',  ( 1.000000000000000000, -1.291538348938060198E-32, 1.054621095516909827E-16 ) ) ;
#1845=PLANE ( 'NONE',  #8363 ) ;
#1848=CARTESIAN_POINT ( 'NONE',  ( 4.000300139189000959, -19.50737899243798879, -12.52892449124999885 ) ) ;
#1862=CARTESIAN_POINT ( 'NONE',  ( -7.681929635180895666, -48.34577715838007350, -7.192553627470831046 ) ) ;
#1872=ORIENTED_EDGE ( 'NONE', *, *, #12630, .F. ) ;
#1874=CARTESIAN_POINT ( 'NONE',  ( -15.49969986081099904, -44.50737899243799944, -109.5506571639849938 ) ) ;
#1876=( BOUNDED_CURVE ( )  B_SPLINE_CURVE ( 3, ( #237, #3751, #8408, #5957 ),
 .UNSPECIFIED., .F., .T. ) 
 B_SPLINE_CURVE_WITH_KNOTS ( ( 4, 4 ),
 ( 0.000000000000000000, 1.570796326794893893 ),
 .UNSPECIFIED. ) 
 CURVE ( )  GEOMETRIC_REPRESENTATION_ITEM ( )  RATIONAL_B_SPLINE_CURVE ( ( 1.000000000000000000, 0.8047378541243654926, 0.8047378541243654926, 1.000000000000000000 ) ) 
 REPRESENTATION_ITEM ( '' )  );
#1884=DIRECTION ( 'NONE',  ( 1.000000000000000000, -1.291538348938060198E-32, 1.054621095516909827E-16 ) ) ;
#1892=CARTESIAN_POINT ( 'NONE',  ( -15.49969986081099904, -52.50737899243799944, 57.00231026484399166 ) ) ;
#1900=CARTESIAN_POINT ( 'NONE',  ( -15.49969986081099904, -27.00737899243800300, -13.49768973515600301 ) ) ;
#1904=CARTESIAN_POINT ( 'NONE',  ( -7.730254068284388325, -46.40242140125007353, -2.999336575030471685 ) ) ;
#1918=CARTESIAN_POINT ( 'NONE',  ( -8.371409249847948431, -48.14116718798079120, 46.40142299527308012 ) ) ;
#1921=CARTESIAN_POINT ( 'NONE',  ( -15.49969986081099904, -13.50737899243800122, 51.00231026484400587 ) ) ;
#1922=FACE_OUTER_BOUND ( 'NONE', #12201, .T. ) ;
#1936=DIRECTION ( 'NONE',  ( -1.734723475976808080E-16, 0.000000000000000000, 1.000000000000000000 ) ) ;
#1958=DIRECTION ( 'NONE',  ( -1.734723475976805615E-16, 0.000000000000000000, 1.000000000000000000 ) ) ;
#1970=DIRECTION ( 'NONE',  ( 0.000000000000000000, 0.000000000000000000, -1.000000000000000000 ) ) ;
#1982=DIRECTION ( 'NONE',  ( -1.000000000000000000, -3.839882694219489529E-17, 0.000000000000000000 ) ) ;
#1990=CARTESIAN_POINT ( 'NONE',  ( -5.499699860811003482, -46.50737899243799944, 44.50231026484399877 ) ) ;
#2005=CARTESIAN_POINT ( 'NONE',  ( -5.499699860811004370, -46.50737899243799944, 44.50231026484399877 ) ) ;
#2012=ADVANCED_FACE ( 'NONE', ( #5620 ), #2416, .T. ) ;
#2018=CARTESIAN_POINT ( 'NONE',  ( 2.500300139188999182, -42.00737899243800655, 52.39987856403599409 ) ) ;
#2019=ORIENTED_EDGE ( 'NONE', *, *, #11672, .T. ) ;
#2022=ORIENTED_EDGE ( 'NONE', *, *, #10197, .F. ) ;
#2025=AXIS2_PLACEMENT_3D ( 'NONE', #2302, #10326, #4523 ) ;
#2026=DIRECTION ( 'NONE',  ( 0.000000000000000000, 0.000000000000000000, 1.000000000000000000 ) ) ;
#2027=DIRECTION ( 'NONE',  ( 0.000000000000000000, 1.000000000000000000, 1.224646799147350002E-16 ) ) ;
#2031=DIRECTION ( 'NONE',  ( 1.054621095516909827E-16, 0.000000000000000000, -1.000000000000000000 ) ) ;
#2034=CARTESIAN_POINT ( 'NONE',  ( -7.753733168396166775, -46.50737899243799944, 42.00231026484399166 ) ) ;
#2043=DIRECTION ( 'NONE',  ( 0.000000000000000000, 0.000000000000000000, 1.000000000000000000 ) ) ;
#2045=CARTESIAN_POINT ( 'NONE',  ( -15.49969986081099904, -27.00737899243800300, -5.497689735156002122 ) ) ;
#2049=CARTESIAN_POINT ( 'NONE',  ( -7.553613233656760073, -48.84439576093267021, 20.40192502283242959 ) ) ;
#2056=CARTESIAN_POINT ( 'NONE',  ( -7.509061791769728877, -44.91935217387478474, -3.566842261944418890 ) ) ;
#2058=LINE ( 'NONE', #1206, #13789 ) ;
#2059=EDGE_CURVE ( 'NONE', #11803, #2347, #9290, .T. ) ;
#2062=ORIENTED_EDGE ( 'NONE', *, *, #5233, .T. ) ;
#2066=CARTESIAN_POINT ( 'NONE',  ( -11.94576515372786751, -51.69378783610798678, 56.83668549888485444 ) ) ;
#2072=CARTESIAN_POINT ( 'NONE',  ( 2.500300139188999182, -46.50737899243799944, 19.50231026484399877 ) ) ;
#2083=ORIENTED_EDGE ( 'NONE', *, *, #4124, .T. ) ;
#2091=CARTESIAN_POINT ( 'NONE',  ( -7.867938255526238933, -47.21659244687199219, -7.899326032359201832 ) ) ;
#2092=CARTESIAN_POINT ( 'NONE',  ( -18.08104095141683487, -52.09767164165551634, -17.91190622590529102 ) ) ;
#2093=VERTEX_POINT ( 'NONE', #13961 ) ;
#2099=CARTESIAN_POINT ( 'NONE',  ( 2.598755596215367447, -41.01804242336424267, 52.34582402777507326 ) ) ;
#2108=CARTESIAN_POINT ( 'NONE',  ( -7.509081646391243758, -44.91911869546537162, 21.43296569163635112 ) ) ;
#2117=CARTESIAN_POINT ( 'NONE',  ( -23.49969986081100259, -44.24330093701085787, 56.13904046828874073 ) ) ;
#2123=CIRCLE ( 'NONE', #12879, 8.000000000000000000 ) ;
#2126=VERTEX_POINT ( 'NONE', #1494 ) ;
#2129=B_SPLINE_CURVE_WITH_KNOTS ( 'NONE', 3,
 ( #11939, #9713, #7409, #1456, #6103, #12092 ),
 .UNSPECIFIED., .F., .F.,
 ( 4, 2, 4 ),
 ( 0.7880782322772789117, 0.8940391161386394003, 1.000000000000000000 ),
 .UNSPECIFIED. ) ;
#2130=DIRECTION ( 'NONE',  ( 0.000000000000000000, -1.000000000000000000, -1.224646799147350002E-16 ) ) ;
#2131=CIRCLE ( 'NONE', #1633, 3.000000000000002665 ) ;
#2135=CARTESIAN_POINT ( 'NONE',  ( -7.753733168396170328, -46.50737899243799944, 47.00231026484399877 ) ) ;
#2137=B_SPLINE_CURVE_WITH_KNOTS ( 'NONE', 3,
 ( #885, #6678, #5836, #15102, #14038, #5613, #5691, #6750, #961, #15027, #10514, #4630, #4477, #9203, #2108, #3477, #8133, #2259, #6971, #42, #4709, #9056, #2182 ),
 .UNSPECIFIED., .F., .F.,
 ( 4, 2, 2, 2, 2, 2, 2, 2, 1, 1, 1, 2, 4 ),
 ( 0.1210918566152707487, 0.1627725786707973910, 0.2044533007263240609, 0.2878147448373775674, 0.4545376330594838032, 0.5378990771705385310, 0.5587394381983011860, 0.5613444833267742240, 0.5639495284552472620, 0.5691596187121935602, 0.5795797992260810494, 0.6212605212816443290, 0.7879834095039132125 ),
 .UNSPECIFIED. ) ;
#2139=CARTESIAN_POINT ( 'NONE',  ( -11.48672836878686532, -51.44777436587664710, 56.78953867381472520 ) ) ;
#2141=EDGE_CURVE ( 'NONE', #5522, #4357, #99, .T. ) ;
#2162=CARTESIAN_POINT ( 'NONE',  ( 0.8918609567539013128, -25.75737899243799944, -17.99768973515599768 ) ) ;
#2167=ORIENTED_EDGE ( 'NONE', *, *, #5276, .F. ) ;
#2174=ORIENTED_EDGE ( 'NONE', *, *, #3341, .T. ) ;
#2179=VECTOR ( 'NONE', #4222, 1000.000000000000000 ) ;
#2181=CARTESIAN_POINT ( 'NONE',  ( -15.49969986081099904, -37.00737899243799944, 19.50231026484399877 ) ) ;
#2182=CARTESIAN_POINT ( 'NONE',  ( -7.501950027729723303, -44.50597529135383468, 20.99749114769749880 ) ) ;
#2185=VERTEX_POINT ( 'NONE', #202 ) ;
#2191=ORIENTED_EDGE ( 'NONE', *, *, #9300, .F. ) ;
#2211=PLANE ( 'NONE',  #12068 ) ;
#2218=CARTESIAN_POINT ( 'NONE',  ( -7.512805849530849400, -44.04964101872670312, 19.04457229113268113 ) ) ;
#2224=ORIENTED_EDGE ( 'NONE', *, *, #8966, .F. ) ;
#2227=CARTESIAN_POINT ( 'NONE',  ( -15.49969986081099904, -26.50737899243800300, 19.50231026484400232 ) ) ;
#2238=CARTESIAN_POINT ( 'NONE',  ( -23.49969986081100615, -44.76879304137393234, -17.13441993860073254 ) ) ;
#2252=ADVANCED_FACE ( 'NONE', ( #13500 ), #8669, .T. ) ;
#2254=AXIS2_PLACEMENT_3D ( 'NONE', #5292, #4071, #13196 ) ;
#2259=CARTESIAN_POINT ( 'NONE',  ( -7.508535857682161030, -44.90886896333648792, 21.42449717988529656 ) ) ;
#2263=CARTESIAN_POINT ( 'NONE',  ( -7.499699860810999041, -44.50737899243799944, 43.00231026484400587 ) ) ;
#2266=B_SPLINE_CURVE_WITH_KNOTS ( 'NONE', 3,
 ( #13174, #6030, #4909, #397, #9716, #13248, #7411, #14605, #10078, #13393, #761, #12163, #8708, #1678, #2757, #11087, #7703, #5197, #14534, #13466, #8562, #610, #14456, #6407, #1831, #9866, #2973, #6258, #12094, #12239, #8783, #2903, #468, #6477, #1605 ),
 .UNSPECIFIED., .F., .F.,
 ( 4, 2, 2, 2, 2, 2, 2, 2, 2, 1, 1, 2, 2, 2, 1, 1, 1, 2, 2, 4 ),
 ( 0.000000000000000000, 0.06249999999999285294, 0.09374999999998914757, 0.1249999999999854283, 0.1874999999999780176, 0.2187499999999731326, 0.2499999999999682476, 0.3749999999999460432, 0.4374999999999342193, 0.4687499999999275024, 0.4843749999999235056, 0.4921874999999215072, 0.4999999999999195088, 0.6249999999999151790, 0.6874999999999131806, 0.7187499999999130695, 0.7343749999999139577, 0.7421874999999155120, 0.7499999999999169553, 1.000000000000000000 ),
 .UNSPECIFIED. ) ;
#2273=CARTESIAN_POINT ( 'NONE',  ( -15.49969986081099371, -36.50737899243799944, -17.99768973515599768 ) ) ;
#2278=EDGE_CURVE ( 'NONE', #10020, #234, #720, .T. ) ;
#2300=CARTESIAN_POINT ( 'NONE',  ( -38.49969986081099904, -37.00737899243799944, 49.12071670408379731 ) ) ;
#2302=CARTESIAN_POINT ( 'NONE',  ( -5.499699860810998153, -46.50737899243799944, -5.497689735156003010 ) ) ;
#2306=DIRECTION ( 'NONE',  ( -1.000000000000000000, 0.000000000000000000, 0.000000000000000000 ) ) ;
#2320=CARTESIAN_POINT ( 'NONE',  ( -23.48691887691489910, -45.03073692993354626, -17.13721805342403570 ) ) ;
#2328=CARTESIAN_POINT ( 'NONE',  ( 3.941853951887407614, -38.49305635557872307, 51.56919050049003772 ) ) ;
#2330=CARTESIAN_POINT ( 'NONE',  ( -20.10554184627359220, -22.38357163673832417, 56.71843902453247921 ) ) ;
#2347=VERTEX_POINT ( 'NONE', #4084 ) ;
#2355=CARTESIAN_POINT ( 'NONE',  ( -15.42469993581076970, -23.50709773904532085, 57.00223526491900117 ) ) ;
#2357=CARTESIAN_POINT ( 'NONE',  ( -23.49969986081101325, -39.82108749142274462, -10.18398123617126316 ) ) ;
#2376=CARTESIAN_POINT ( 'NONE',  ( -7.707857435416944014, -48.23250629231415587, -7.308525619473091872 ) ) ;
#2377=CARTESIAN_POINT ( 'NONE',  ( -36.19566670804134390, -37.55864118711514976, 50.77578715576750312 ) ) ;
#2385=ORIENTED_EDGE ( 'NONE', *, *, #9612, .T. ) ;
#2386=EDGE_CURVE ( 'NONE', #10391, #3246, #2131, .T. ) ;
#2389=VECTOR ( 'NONE', #4340, 1000.000000000000000 ) ;
#2396=CARTESIAN_POINT ( 'NONE',  ( -15.49969986081099904, -13.50737899243800122, 48.00231026484399877 ) ) ;
#2397=DIRECTION ( 'NONE',  ( 0.000000000000000000, -1.000000000000000000, -1.224646799147350002E-16 ) ) ;
#2399=CARTESIAN_POINT ( 'NONE',  ( 5.481341784370953540, -37.42264482913269319, -11.58109560547579875 ) ) ;
#2406=CARTESIAN_POINT ( 'NONE',  ( -19.27885705962587792, -22.80299515092378115, 56.81857148815599601 ) ) ;
#2416=PLANE ( 'NONE',  #13052 ) ;
#2418=VERTEX_POINT ( 'NONE', #2018 ) ;
#2428=VECTOR ( 'NONE', #5035, 1000.000000000000000 ) ;
#2444=DIRECTION ( 'NONE',  ( 0.000000000000000000, 0.000000000000000000, -1.000000000000000000 ) ) ;
#2450=CARTESIAN_POINT ( 'NONE',  ( -37.48126337154804588, -37.10904096101435812, 49.88474612916678552 ) ) ;
#2455=VERTEX_POINT ( 'NONE', #6891 ) ;
#2459=EDGE_CURVE ( 'NONE', #6722, #9646, #12146, .T. ) ;
#2470=CARTESIAN_POINT ( 'NONE',  ( 5.849866904682269997, -37.28744580235388639, -11.32700113113168250 ) ) ;
#2474=CARTESIAN_POINT ( 'NONE',  ( 5.699973058922845226, -37.34275670915351952, 50.43488819123945888 ) ) ;
#2480=VECTOR ( 'NONE', #10094, 1000.000000000000000 ) ;
#2482=CARTESIAN_POINT ( 'NONE',  ( -7.510313973563612855, -44.09312080494210306, 20.19350477440718805 ) ) ;
#2483=DIRECTION ( 'NONE',  ( -1.000000000000000000, 0.000000000000000000, 0.000000000000000000 ) ) ;
#2486=CARTESIAN_POINT ( 'NONE',  ( -23.49969986081101325, -39.82108749142274462, -0.8113982341407446341 ) ) ;
#2490=SURFACE_SIDE_STYLE ('',( #1194 ) ) ;
#2495=EDGE_CURVE ( 'NONE', #7103, #11225, #11159, .T. ) ;
#2509=VERTEX_POINT ( 'NONE', #4848 ) ;
#2512=DIRECTION ( 'NONE',  ( 1.000000000000000000, -1.291538348938060198E-32, 1.054621095516909827E-16 ) ) ;
#2516=AXIS2_PLACEMENT_3D ( 'NONE', #2227, #9176, #7872 ) ;
#2520=CARTESIAN_POINT ( 'NONE',  ( -23.49969986081099904, -19.50737899243800300, 51.00231026484400587 ) ) ;
#2522=EDGE_LOOP ( 'NONE', ( #577, #10692, #12091, #12428 ) ) ;
#2523=CARTESIAN_POINT ( 'NONE',  ( -8.994852257141582541, -49.17162665769217966, -17.42950165714590227 ) ) ;
#2537=CYLINDRICAL_SURFACE ( 'NONE', #13422, 4.999999999999997335 ) ;
#2553=DIRECTION ( 'NONE',  ( 0.000000000000000000, 0.000000000000000000, 1.000000000000000000 ) ) ;
#2555=CARTESIAN_POINT ( 'NONE',  ( -16.28220704778704686, -23.50179128533422102, 57.00082024756494548 ) ) ;
#2556=EDGE_CURVE ( 'NONE', #818, #1516, #5737, .T. ) ;
#2562=CARTESIAN_POINT ( 'NONE',  ( -7.499699427612007696, -49.00737706678064853, -5.512197160768672610 ) ) ;
#2570=CARTESIAN_POINT ( 'NONE',  ( -20.38418912502062952, -38.15003195939497260, 56.68542173094085257 ) ) ;
#2572=CARTESIAN_POINT ( 'NONE',  ( -7.551842794993419261, -43.45459616270409953, -17.14591884814140954 ) ) ;
#2575=VECTOR ( 'NONE', #863, 1000.000000000000000 ) ;
#2578=CARTESIAN_POINT ( 'NONE',  ( -9.151507943007304746, -21.23407436738225940, 56.46085224906951083 ) ) ;
#2579=B_SPLINE_CURVE_WITH_KNOTS ( 'NONE', 3,
 ( #1348, #10674, #206, #8820, #13434, #7372, #576, #1797, #724, #6448, #14497, #10978, #1643, #504, #12355, #9830, #8526, #6224, #6299, #2795, #5241, #13215 ),
 .UNSPECIFIED., .F., .F.,
 ( 4, 2, 2, 2, 2, 2, 2, 2, 2, 2, 4 ),
 ( 0.000000000000000000, 0.001575908489663656407, 0.002363862734495489597, 0.003151816979327322788, 0.004727725468990988736, 0.006303633958654655117, 0.007091588203486492645, 0.007879542448318330172, 0.009455450937982013901, 0.01103135942764569936, 0.01260726791730938309 ),
 .UNSPECIFIED. ) ;
#2593=CARTESIAN_POINT ( 'NONE',  ( -15.49969986081099904, -27.00737899243800300, 19.50231026484400587 ) ) ;
#2613=DIRECTION ( 'NONE',  ( 1.000000000000000000, 0.000000000000000000, 0.000000000000000000 ) ) ;
#2614=EDGE_CURVE ( 'NONE', #13213, #13055, #7871, .T. ) ;
#2630=VECTOR ( 'NONE', #7244, 1000.000000000000000 ) ;
#2638=EDGE_LOOP ( 'NONE', ( #10828, #698, #9288, #112, #12732, #11330, #7445, #12382 ) ) ;
#2646=CARTESIAN_POINT ( 'NONE',  ( -18.08313173950247688, -36.91805501818645752, 56.91633806427406483 ) ) ;
#2656=CARTESIAN_POINT ( 'NONE',  ( -15.49969986081099016, -57.00737899243800655, 27.50231026484399521 ) ) ;
#2658=VERTEX_POINT ( 'NONE', #14292 ) ;
#2662=DIRECTION ( 'NONE',  ( 0.7071067811865475727, 0.7071067811865475727, 1.202263280131018653E-17 ) ) ;
#2668=DIRECTION ( 'NONE',  ( 0.000000000000000000, 1.224646799147350002E-16, -1.000000000000000000 ) ) ;
#2674=ORIENTED_EDGE ( 'NONE', *, *, #13007, .F. ) ;
#2688=CARTESIAN_POINT ( 'NONE',  ( -15.49969986081099371, -19.50737899243800300, -17.99768973515599768 ) ) ;
#2692=EDGE_CURVE ( 'NONE', #1229, #12928, #3885, .T. ) ;
#2701=DIRECTION ( 'NONE',  ( -3.632077277826439854E-16, 1.000000000000000000, 0.000000000000000000 ) ) ;
#2702=VERTEX_POINT ( 'NONE', #5478 ) ;
#2707=EDGE_CURVE ( 'NONE', #11105, #4357, #894, .T. ) ;
#2713=ORIENTED_EDGE ( 'NONE', *, *, #5690, .T. ) ;
#2714=CARTESIAN_POINT ( 'NONE',  ( -23.49969986081101325, -49.19367049345325427, 14.81601876382875105 ) ) ;
#2720=ORIENTED_EDGE ( 'NONE', *, *, #6346, .F. ) ;
#2722=CARTESIAN_POINT ( 'NONE',  ( -15.49969986081099904, -57.00737899243800655, -5.497689735156002122 ) ) ;
#2744=CARTESIAN_POINT ( 'NONE',  ( -7.844836682715777165, -47.42038978965553042, 17.17387271121222270 ) ) ;
#2745=VECTOR ( 'NONE', #8372, 1000.000000000000000 ) ;
#2749=DIRECTION ( 'NONE',  ( 0.000000000000000000, -1.000000000000000000, -1.224646799147350002E-16 ) ) ;
#2753=CARTESIAN_POINT ( 'NONE',  ( -33.63837922572173511, -40.83713880675461638, 52.32362684487226545 ) ) ;
#2754=VERTEX_POINT ( 'NONE', #4287 ) ;
#2757=CARTESIAN_POINT ( 'NONE',  ( -34.27301134323082721, -39.31333522014669057, -12.96100848131858108 ) ) ;
#2769=CIRCLE ( 'NONE', #1788, 37.50000000000000000 ) ;
#2770=DIRECTION ( 'NONE',  ( -1.000000000000000000, -1.291538348938060198E-32, 1.054621095516909827E-16 ) ) ;
#2774=CARTESIAN_POINT ( 'NONE',  ( -34.99969986081099904, -19.50737899243800300, 51.53354502093799994 ) ) ;
#2780=EDGE_CURVE ( 'NONE', #8988, #13722, #13619, .T. ) ;
#2786=CARTESIAN_POINT ( 'NONE',  ( -7.667215781397969998, -48.40529181397006653, -7.124959850448637333 ) ) ;
#2789=CYLINDRICAL_SURFACE ( 'NONE', #8733, 4.999999999999997335 ) ;
#2795=CARTESIAN_POINT ( 'NONE',  ( -23.44796623947610570, -45.55538915506302544, 56.15044716263313518 ) ) ;
#2803=CARTESIAN_POINT ( 'NONE',  ( -12.47873212575276192, -23.04849409689505890, 56.88099131889190119 ) ) ;
#2804=EDGE_CURVE ( 'NONE', #12356, #7103, #12252, .T. ) ;
#2809=CARTESIAN_POINT ( 'NONE',  ( -7.495514965259227225, -43.99345095228513003, -5.653725713467976810 ) ) ;
#2810=VERTEX_POINT ( 'NONE', #851 ) ;
#2814=DIRECTION ( 'NONE',  ( 0.000000000000000000, 0.000000000000000000, 1.000000000000000000 ) ) ;
#2823=CARTESIAN_POINT ( 'NONE',  ( -15.42469986081099442, -23.50709773848280904, 56.85231026484400019 ) ) ;
#2826=CARTESIAN_POINT ( 'NONE',  ( -34.03229764406204794, -39.75996117776632843, 52.10284593195687108 ) ) ;
#2830=ORIENTED_EDGE ( 'NONE', *, *, #6730, .T. ) ;
#2836=CARTESIAN_POINT ( 'NONE',  ( -7.754954776104139746, -46.50766419030464505, -2.997807438439666239 ) ) ;
#2838=ADVANCED_FACE ( 'NONE', ( #2989 ), #4216, .F. ) ;
#2859=AXIS2_PLACEMENT_3D ( 'NONE', #11837, #376, #6163 ) ;
#2860=ORIENTED_EDGE ( 'NONE', *, *, #14251, .F. ) ;
#2875=FACE_BOUND ( 'NONE', #1621, .T. ) ;
#2881=ADVANCED_FACE ( 'NONE', ( #5356 ), #10016, .F. ) ;
#2890=CARTESIAN_POINT ( 'NONE',  ( -7.867938255526322422, -47.21659244687067059, 17.10067396764040737 ) ) ;
#2893=ADVANCED_FACE ( 'NONE', ( #82 ), #998, .F. ) ;
#2902=ORIENTED_EDGE ( 'NONE', *, *, #684, .F. ) ;
#2903=CARTESIAN_POINT ( 'NONE',  ( -36.75660122519333584, -37.32104008884121527, -11.39096713563728258 ) ) ;
#2915=EDGE_CURVE ( 'NONE', #2185, #2996, #5952, .T. ) ;
#2918=CARTESIAN_POINT ( 'NONE',  ( -7.504222113441009867, -44.23130020225004699, 43.45950419441649615 ) ) ;
#2934=LINE ( 'NONE', #12115, #5573 ) ;
#2939=DIRECTION ( 'NONE',  ( -1.000000000000000000, 1.291538348938060198E-32, -1.054621095516909827E-16 ) ) ;
#2964=CARTESIAN_POINT ( 'NONE',  ( -7.667215781397985097, -48.40529181396999547, 17.87504014955130316 ) ) ;
#2969=CARTESIAN_POINT ( 'NONE',  ( -7.754954776104139746, -46.50766419030464505, -2.997807438439666239 ) ) ;
#2973=CARTESIAN_POINT ( 'NONE',  ( -36.26264625145540776, -37.53054613521290150, -11.72591093593669065 ) ) ;
#2976=CARTESIAN_POINT ( 'NONE',  ( -8.992083836518988349, -50.38952316532486009, 25.38445443773086296 ) ) ;
#2989=FACE_OUTER_BOUND ( 'NONE', #14981, .T. ) ;
#2995=CARTESIAN_POINT ( 'NONE',  ( -2.716578225681299141, -32.00737899243799944, 54.75627176226269199 ) ) ;
#2996=VERTEX_POINT ( 'NONE', #2520 ) ;
#2997=ORIENTED_EDGE ( 'NONE', *, *, #3014, .T. ) ;
#3014=EDGE_CURVE ( 'NONE', #2418, #5221, #387, .T. ) ;
#3022=CYLINDRICAL_SURFACE ( 'NONE', #4992, 8.000000000000000000 ) ;
#3036=CYLINDRICAL_SURFACE ( 'NONE', #4460, 8.000000000000000000 ) ;
#3039=SHAPE_DEFINITION_REPRESENTATION ( #542, #410 ) ;
#3040=CARTESIAN_POINT ( 'NONE',  ( -7.654737080345058509, -48.45581950336342913, 21.06873913907410412 ) ) ;
#3055=CARTESIAN_POINT ( 'NONE',  ( -8.552266936091450944, -48.47531820779182254, 46.05263013242581849 ) ) ;
#3057=DIRECTION ( 'NONE',  ( 1.000000000000000000, 0.000000000000000000, 0.000000000000000000 ) ) ;
#3059=CARTESIAN_POINT ( 'NONE',  ( -7.499699860811000818, -44.42718604110348934, 43.10923419995668837 ) ) ;
#3060=EDGE_CURVE ( 'NONE', #12888, #2455, #10704, .T. ) ;
#3064=CARTESIAN_POINT ( 'NONE',  ( -7.499699860810999041, -44.50737899243799944, -109.5506571639849938 ) ) ;
#3077=DIRECTION ( 'NONE',  ( 0.000000000000000000, 1.000000000000000000, 1.224646799147350002E-16 ) ) ;
#3081=ORIENTED_EDGE ( 'NONE', *, *, #12175, .F. ) ;
#3083=EDGE_CURVE ( 'NONE', #11803, #1385, #14653, .T. ) ;
#3089=CARTESIAN_POINT ( 'NONE',  ( 2.539580576486363039, -41.37673382706633873, 52.37835757418703508 ) ) ;
#3091=CARTESIAN_POINT ( 'NONE',  ( -7.794857923030186875, -46.66268402978349883, -7.997689078744453894 ) ) ;
#3097=CARTESIAN_POINT ( 'NONE',  ( -15.49969986081099904, -44.50737899243799944, -109.5506571639849938 ) ) ;
#3098=LINE ( 'NONE', #7757, #5702 ) ;
#3100=EDGE_LOOP ( 'NONE', ( #6231, #13537, #10368, #10274, #7595 ) ) ;
#3116=CARTESIAN_POINT ( 'NONE',  ( -7.600774661673999510, -48.67202872725025031, 20.75559684966261287 ) ) ;
#3128=VERTEX_POINT ( 'NONE', #1900 ) ;
#3130=VECTOR ( 'NONE', #5393, 1000.000000000000000 ) ;
#3133=CARTESIAN_POINT ( 'NONE',  ( -7.499699860810997265, -45.03100262877134696, 56.13904046828873362 ) ) ;
#3134=CARTESIAN_POINT ( 'NONE',  ( -34.99969986081099904, -20.37340439622244048, -12.52892449124999885 ) ) ;
#3137=DIRECTION ( 'NONE',  ( -1.000000000000000000, -3.700743415417187646E-16, 0.000000000000000000 ) ) ;
#3141=CARTESIAN_POINT ( 'NONE',  ( -38.49969986081099904, -37.00737899243799944, -10.11609617439569675 ) ) ;
#3154=CARTESIAN_POINT ( 'NONE',  ( 7.500300139189000070, -37.00737899243799944, 19.50231026484400587 ) ) ;
#3160=ORIENTED_EDGE ( 'NONE', *, *, #13007, .T. ) ;
#3164=ORIENTED_EDGE ( 'NONE', *, *, #2141, .T. ) ;
#3173=CARTESIAN_POINT ( 'NONE',  ( -28.28282149594069850, -32.00737899243799944, -15.75165123257469801 ) ) ;
#3183=B_SPLINE_CURVE_WITH_KNOTS ( 'NONE', 3,
 ( #6426, #1698, #5219, #11183, #14552, #5366, #12484, #14624, #702, #4067 ),
 .UNSPECIFIED., .F., .F.,
 ( 4, 2, 2, 2, 4 ),
 ( 0.2882554882889244441, 0.4355039734903317639, 0.5091282160910374222, 0.5827524586917430804, 0.8772494290945609396 ),
 .UNSPECIFIED. ) ;
#3184=ORIENTED_EDGE ( 'NONE', *, *, #2495, .F. ) ;
#3188=AXIS2_PLACEMENT_3D ( 'NONE', #9436, #5010, #8514 ) ;
#3192=CYLINDRICAL_SURFACE ( 'NONE', #8082, 8.000000000000000000 ) ;
#3193=DIRECTION ( 'NONE',  ( 0.000000000000000000, -1.000000000000000000, -1.224646799147350002E-16 ) ) ;
#3195=CARTESIAN_POINT ( 'NONE',  ( -7.838594959942573936, -47.52544946158244699, 21.80362717976635878 ) ) ;
#3197=CARTESIAN_POINT ( 'NONE',  ( -15.49969986081099016, -52.50737899243799944, 27.50231026484399521 ) ) ;
#3202=EDGE_LOOP ( 'NONE', ( #6388, #12314, #12186, #12035 ) ) ;
#3211=CARTESIAN_POINT ( 'NONE',  ( -7.844606716089023379, -46.83718042189172337, 42.01877877715759269 ) ) ;
#3223=EDGE_LOOP ( 'NONE', ( #7297, #11784, #1458, #12605, #13746, #6701, #5995, #4937, #13540 ) ) ;
#3229=ORIENTED_EDGE ( 'NONE', *, *, #2692, .F. ) ;
#3242=EDGE_LOOP ( 'NONE', ( #4773, #10389 ) ) ;
#3246=VERTEX_POINT ( 'NONE', #603 ) ;
#3259=FACE_OUTER_BOUND ( 'NONE', #13431, .T. ) ;
#3269=ORIENTED_EDGE ( 'NONE', *, *, #9342, .T. ) ;
#3276=CARTESIAN_POINT ( 'NONE',  ( -31.57904533557009330, -52.92803351767890518, -14.44614973369545474 ) ) ;
#3278=VERTEX_POINT ( 'NONE', #6922 ) ;
#3281=AXIS2_PLACEMENT_3D ( 'NONE', #11536, #1058, #5717 ) ;
#3290=CARTESIAN_POINT ( 'NONE',  ( -9.472454833892761883, -49.79350169645305613, 56.51664171905113676 ) ) ;
#3292=CARTESIAN_POINT ( 'NONE',  ( -8.872668239290053549, -48.98891758557466858, 44.15515983234535469 ) ) ;
#3304=ORIENTED_EDGE ( 'NONE', *, *, #12542, .T. ) ;
#3311=EDGE_CURVE ( 'NONE', #6735, #12112, #4286, .T. ) ;
#3313=CARTESIAN_POINT ( 'NONE',  ( -21.85949554531645234, -49.38834405300886488, -17.45563142244668953 ) ) ;
#3331=DIRECTION ( 'NONE',  ( 0.000000000000000000, 0.000000000000000000, -1.000000000000000000 ) ) ;
#3335=LINE ( 'NONE', #6839, #9339 ) ;
#3336=CARTESIAN_POINT ( 'NONE',  ( -20.78983891441731302, -38.48355218851715875, -17.62454701498858256 ) ) ;
#3340=DIRECTION ( 'NONE',  ( 0.000000000000000000, 1.850371707708594316E-16, -1.000000000000000000 ) ) ;
#3341=EDGE_CURVE ( 'NONE', #11671, #855, #12844, .T. ) ;
#3350=CYLINDRICAL_SURFACE ( 'NONE', #3281, 8.000000000000000000 ) ;
#3380=CARTESIAN_POINT ( 'NONE',  ( -30.62513859619093637, -27.95036676736707548, 53.90694524323490100 ) ) ;
#3399=CARTESIAN_POINT ( 'NONE',  ( -21.63983770886135005, -21.40953461391054802, 56.49919483392252317 ) ) ;
#3411=VECTOR ( 'NONE', #14729, 1000.000000000000000 ) ;
#3424=VERTEX_POINT ( 'NONE', #2656 ) ;
#3426=CARTESIAN_POINT ( 'NONE',  ( -5.499699860810998153, -46.50737899243799944, -5.497689735156003010 ) ) ;
#3434=EDGE_CURVE ( 'NONE', #7373, #12214, #4095, .T. ) ;
#3435=AXIS2_PLACEMENT_3D ( 'NONE', #10644, #1389, #14089 ) ;
#3439=DIRECTION ( 'NONE',  ( -1.000000000000000000, -3.632077277826439854E-16, 0.000000000000000000 ) ) ;
#3445=ORIENTED_EDGE ( 'NONE', *, *, #3900, .T. ) ;
#3448=ORIENTED_EDGE ( 'NONE', *, *, #3014, .F. ) ;
#3461=CARTESIAN_POINT ( 'NONE',  ( 6.268676098693725329, -37.15669500878450293, -11.03356574139771418 ) ) ;
#3473=CIRCLE ( 'NONE', #13978, 3.000000000000002665 ) ;
#3477=CARTESIAN_POINT ( 'NONE',  ( -7.508989031724891738, -44.91746444383585413, 21.43160362669583563 ) ) ;
#3486=CARTESIAN_POINT ( 'NONE',  ( -23.49969986081099904, -43.98440953699977740, -17.13441993860073609 ) ) ;
#3489=CARTESIAN_POINT ( 'NONE',  ( -8.559440489995196799, -40.49367064263154248, -17.35106608438774956 ) ) ;
#3517=CARTESIAN_POINT ( 'NONE',  ( -7.836123178633707553, -47.48973556348613556, -7.797900083227910173 ) ) ;
#3526=VERTEX_POINT ( 'NONE', #5131 ) ;
#3530=FACE_OUTER_BOUND ( 'NONE', #12405, .T. ) ;
#3533=CARTESIAN_POINT ( 'NONE',  ( -1.425463962227826897, -54.93314309385483085, -15.32525311590548434 ) ) ;
#3540=ORIENTED_EDGE ( 'NONE', *, *, #8696, .T. ) ;
#3541=CARTESIAN_POINT ( 'NONE',  ( 5.815276763445654140, -37.29975643136119601, -11.35092641676986780 ) ) ;
#3549=CARTESIAN_POINT ( 'NONE',  ( -20.04324321135802833, -22.41562731333683089, 56.72605870807743145 ) ) ;
#3557=FACE_OUTER_BOUND ( 'NONE', #12087, .T. ) ;
#3566=CARTESIAN_POINT ( 'NONE',  ( -11.49146427699059814, -37.56416174903810656, -17.78544053839978289 ) ) ;
#3576=VECTOR ( 'NONE', #3439, 1000.000000000000000 ) ;
#3584=DIRECTION ( 'NONE',  ( 0.000000000000000000, 0.000000000000000000, -1.000000000000000000 ) ) ;
#3588=AXIS2_PLACEMENT_3D ( 'NONE', #1990, #6863, #11550 ) ;
#3589=LINE ( 'NONE', #12939, #608 ) ;
#3594=CARTESIAN_POINT ( 'NONE',  ( -3.499699860810999041, -57.00737899243800655, -16.02584758213710003 ) ) ;
#3596=EDGE_LOOP ( 'NONE', ( #10331, #1203, #8201, #6576, #5146, #9852 ) ) ;
#3598=ORIENTED_EDGE ( 'NONE', *, *, #12152, .F. ) ;
#3599=VECTOR ( 'NONE', #12995, 1000.000000000000000 ) ;
#3614=CARTESIAN_POINT ( 'NONE',  ( -7.499699860810998153, -44.50737899243799944, 56.13904046828873362 ) ) ;
#3617=ORIENTED_EDGE ( 'NONE', *, *, #1798, .F. ) ;
#3620=CARTESIAN_POINT ( 'NONE',  ( 2.818822887961262236, -40.24903322726662225, 52.22360476062456769 ) ) ;
#3632=CARTESIAN_POINT ( 'NONE',  ( -7.512805849530849400, -44.04964101872660365, 19.96004823855532706 ) ) ;
#3636=CARTESIAN_POINT ( 'NONE',  ( -15.49969986081099194, -52.50737899243800655, 11.50231026484399521 ) ) ;
#3642=ORIENTED_EDGE ( 'NONE', *, *, #4125, .F. ) ;
#3653=CIRCLE ( 'NONE', #3907, 8.000000000000000000 ) ;
#3665=DIRECTION ( 'NONE',  ( 0.000000000000000000, -1.000000000000000000, -1.224646799147350002E-16 ) ) ;
#3667=DIRECTION ( 'NONE',  ( 0.000000000000000000, 0.000000000000000000, 1.000000000000000000 ) ) ;
#3671=CIRCLE ( 'NONE', #11001, 10.00000000000000000 ) ;
#3674=CARTESIAN_POINT ( 'NONE',  ( -9.661154126855418411, -49.98269403727269378, -17.54085436190861458 ) ) ;
#3691=EDGE_CURVE ( 'NONE', #4357, #12241, #12024, .T. ) ;
#3693=CARTESIAN_POINT ( 'NONE',  ( 2.660328366240848563, -40.75169664998565366, -13.30720238894809349 ) ) ;
#3694=VERTEX_POINT ( 'NONE', #11315 ) ;
#3718=CARTESIAN_POINT ( 'NONE',  ( -7.706583154360178156, -42.68076247385797473, -17.17902169384817057 ) ) ;
#3724=CARTESIAN_POINT ( 'NONE',  ( -7.593867891459233910, -45.75082787501852977, 17.08720858567314238 ) ) ;
#3733=EDGE_CURVE ( 'NONE', #13947, #13156, #4109, .T. ) ;
#3736=CARTESIAN_POINT ( 'NONE',  ( -7.497191992632178170, -44.39045585651064840, -6.841238297419723224 ) ) ;
#3748=CARTESIAN_POINT ( 'NONE',  ( -11.27121226320114644, -51.30363337802549495, -17.75917625400039057 ) ) ;
#3751=CARTESIAN_POINT ( 'NONE',  ( -20.18599136182623965, -52.50737899243802786, 2.502310264844031185 ) ) ;
#3774=EDGE_LOOP ( 'NONE', ( #13158, #5808 ) ) ;
#3779=CARTESIAN_POINT ( 'NONE',  ( -17.02073322366946684, -23.42091518255481475, 56.97733164403681627 ) ) ;
#3785=CARTESIAN_POINT ( 'NONE',  ( -7.499960972858381147, -49.00661531336379539, -5.561496955626357597 ) ) ;
#3794=ORIENTED_EDGE ( 'NONE', *, *, #6847, .F. ) ;
#3795=CARTESIAN_POINT ( 'NONE',  ( -7.924984455289715513, -41.92032950385904400, -17.22478920316331852 ) ) ;
#3796=EDGE_CURVE ( 'NONE', #14198, #10750, #5665, .T. ) ;
#3798=CARTESIAN_POINT ( 'NONE',  ( -9.290890585402740598, -21.34661493808534516, 56.48450469233716120 ) ) ;
#3803=CARTESIAN_POINT ( 'NONE',  ( -5.499699860810997265, -46.50737899243799944, -5.497689735156003010 ) ) ;
#3805=CARTESIAN_POINT ( 'NONE',  ( -7.497885806132468467, -44.50611869254105102, 18.00659976627173720 ) ) ;
#3811=FACE_OUTER_BOUND ( 'NONE', #7617, .T. ) ;
#3815=CARTESIAN_POINT ( 'NONE',  ( -15.49969986081099194, -57.00737899243800655, 19.50231026484399521 ) ) ;
#3816=AXIS2_PLACEMENT_3D ( 'NONE', #8018, #11696, #9246 ) ;
#3819=CARTESIAN_POINT ( 'NONE',  ( -34.28383802683607939, -39.31204358973022295, 51.95868366853013498 ) ) ;
#3874=CARTESIAN_POINT ( 'NONE',  ( -7.959143533992851793, -20.11997055668047096, 56.24285220617511527 ) ) ;
#3880=VERTEX_POINT ( 'NONE', #151 ) ;
#3881=B_SPLINE_CURVE_WITH_KNOTS ( 'NONE', 3,
 ( #6450, #13583, #578, #11133, #5244, #649, #7747, #5313, #4169, #14220, #7896, #13655, #11277, #5533, #10120, #5760, #14945, #13804, #14876, #10279, #13726, #11430, #4320, #7815, #6827, #11356 ),
 .UNSPECIFIED., .F., .F.,
 ( 4, 2, 2, 2, 2, 2, 2, 2, 2, 2, 2, 2, 4 ),
 ( 0.02522177263268702771, 0.02600995928983864530, 0.02679814594699025943, 0.02837451926129350155, 0.02916270591844511567, 0.02995089257559673326, 0.03152726588989995804, 0.03231545254705157216, 0.03310363920420318629, 0.03389182586135480041, 0.03468001251850641453, 0.03625638583280965666, 0.03783275914711289878 ),
 .UNSPECIFIED. ) ;
#3884=CARTESIAN_POINT ( 'NONE',  ( -7.502372241906894779, -44.29399517289605370, 18.32448191336956000 ) ) ;
#3885=LINE ( 'NONE', #9695, #7241 ) ;
#3890=DIRECTION ( 'NONE',  ( 1.000000000000000000, 0.000000000000000000, 0.000000000000000000 ) ) ;
#3894=CARTESIAN_POINT ( 'NONE',  ( -7.506424547597140950, -48.98717474752370293, 19.17796694551992687 ) ) ;
#3898=CARTESIAN_POINT ( 'NONE',  ( -7.499699860810997265, -45.03775106554863328, -17.13441993860075030 ) ) ;
#3899=CARTESIAN_POINT ( 'NONE',  ( -34.67966921736225316, -38.76197583040457317, 51.72704121311384995 ) ) ;
#3900=EDGE_CURVE ( 'NONE', #6722, #13722, #9238, .T. ) ;
#3907=AXIS2_PLACEMENT_3D ( 'NONE', #2722, #13143, #285 ) ;
#3908=EDGE_CURVE ( 'NONE', #3526, #9567, #10392, .T. ) ;
#3910=CARTESIAN_POINT ( 'NONE',  ( -15.49969986081099904, -13.50737899243800122, 48.00231026484399877 ) ) ;
#3915=CARTESIAN_POINT ( 'NONE',  ( -7.510307729924003084, -44.09336537972112779, 43.83865520846783426 ) ) ;
#3936=EDGE_LOOP ( 'NONE', ( #10642, #11417, #10270, #13817 ) ) ;
#3950=FACE_OUTER_BOUND ( 'NONE', #9390, .T. ) ;
#3955=AXIS2_PLACEMENT_3D ( 'NONE', #7353, #6207, #6430 ) ;
#3956=EDGE_CURVE ( 'NONE', #12928, #818, #4659, .T. ) ;
#3962=CARTESIAN_POINT ( 'NONE',  ( -7.886584594865169606, -46.96511696614940234, 21.96004823855531640 ) ) ;
#3963=VECTOR ( 'NONE', #14471, 1000.000000000000000 ) ;
#3966=EDGE_CURVE ( 'NONE', #1260, #6753, #10102, .T. ) ;
#3967=CARTESIAN_POINT ( 'NONE',  ( -7.797100586692807589, -47.75470106918052693, 17.33567862706513552 ) ) ;
#3976=DIRECTION ( 'NONE',  ( 0.000000000000000000, -1.000000000000000000, -1.224646799147350002E-16 ) ) ;
#3983=CARTESIAN_POINT ( 'NONE',  ( 2.500300139189001847, -46.50737899243799944, -5.497689735156002122 ) ) ;
#3990=CARTESIAN_POINT ( 'NONE',  ( -7.514630092986283039, -44.01837396645046141, 44.23252331109035396 ) ) ;
#3992=AXIS2_PLACEMENT_3D ( 'NONE', #5323, #12439, #1958 ) ;
#3996=ORIENTED_EDGE ( 'NONE', *, *, #177, .F. ) ;
#4002=CIRCLE ( 'NONE', #10839, 2.499999999999999556 ) ;
#4012=DIRECTION ( 'NONE',  ( 0.000000000000000000, -1.000000000000000000, -1.224646799147350002E-16 ) ) ;
#4013=CARTESIAN_POINT ( 'NONE',  ( 2.500300139188999182, -51.00737899243799944, 19.50231026484398456 ) ) ;
#4014=ORIENTED_EDGE ( 'NONE', *, *, #9202, .F. ) ;
#4015=ORIENTED_EDGE ( 'NONE', *, *, #13272, .T. ) ;
#4016=CIRCLE ( 'NONE', #12572, 2.499999999999998668 ) ;
#4030=DIRECTION ( 'NONE',  ( 0.000000000000000000, -1.000000000000000000, -1.224646799147350002E-16 ) ) ;
#4034=ORIENTED_EDGE ( 'NONE', *, *, #11569, .T. ) ;
#4038=CARTESIAN_POINT ( 'NONE',  ( -7.886584594865190034, -46.96511696614940234, 17.04457229113261718 ) ) ;
#4041=VECTOR ( 'NONE', #3667, 1000.000000000000000 ) ;
#4043=ADVANCED_FACE ( 'NONE', ( #5385 ), #11922, .F. ) ;
#4045=CARTESIAN_POINT ( 'NONE',  ( -11.90127153857805453, -52.50737899243803497, -13.49768973515603498 ) ) ;
#4048=CARTESIAN_POINT ( 'NONE',  ( 4.000300139189000959, -20.37340439622242982, -17.99768973515599768 ) ) ;
#4051=LINE ( 'NONE', #6334, #7636 ) ;
#4065=LINE ( 'NONE', #8724, #9570 ) ;
#4067=CARTESIAN_POINT ( 'NONE',  ( -7.754798889200088752, -46.50763646577239285, -7.996864293225370623 ) ) ;
#4071=DIRECTION ( 'NONE',  ( 0.000000000000000000, -1.000000000000000000, -1.224646799147350002E-16 ) ) ;
#4072=EDGE_LOOP ( 'NONE', ( #762, #1587 ) ) ;
#4081=PLANE ( 'NONE',  #10954 ) ;
#4084=CARTESIAN_POINT ( 'NONE',  ( -15.49969986081099904, -57.00737899243800655, -13.49768973515600301 ) ) ;
#4087=EDGE_CURVE ( 'NONE', #8099, #2658, #5162, .T. ) ;
#4088=CARTESIAN_POINT ( 'NONE',  ( -23.49969986081099904, -44.50737899243799944, -5.497689735156002122 ) ) ;
#4090=AXIS2_PLACEMENT_3D ( 'NONE', #14659, #11067, #589 ) ;
#4095=B_SPLINE_CURVE_WITH_KNOTS ( 'NONE', 3,
 ( #6158, #14131, #8460, #14361, #8612, #8538, #7225, #3724, #9535, #8380 ),
 .UNSPECIFIED., .F., .F.,
 ( 4, 2, 2, 2, 4 ),
 ( 0.2880475688081467478, 0.4353390005973231114, 0.5089847164919113487, 0.5826304323864994750, 0.8772132959648567541 ),
 .UNSPECIFIED. ) ;
#4103=CARTESIAN_POINT ( 'NONE',  ( -15.57469986081333424, -26.50737899243800300, 57.00223526477140013 ) ) ;
#4109=( BOUNDED_CURVE ( )  B_SPLINE_CURVE ( 3, ( #11164, #2976, #687, #6559 ),
 .UNSPECIFIED., .F., .T. ) 
 B_SPLINE_CURVE_WITH_KNOTS ( ( 4, 4 ),
 ( 5.024656459356720006, 6.283185307179586232 ),
 .UNSPECIFIED. ) 
 CURVE ( )  GEOMETRIC_REPRESENTATION_ITEM ( )  RATIONAL_B_SPLINE_CURVE ( ( 1.000000000000000000, 0.8723071003127500500, 0.8723071003127500500, 1.000000000000000000 ) ) 
 REPRESENTATION_ITEM ( '' )  );
#4110=CARTESIAN_POINT ( 'NONE',  ( -15.49969986081099194, -52.50737899243800655, 11.50231026484399521 ) ) ;
#4112=LINE ( 'NONE', #12078, #1032 ) ;
#4124=EDGE_CURVE ( 'NONE', #3694, #1385, #6970, .T. ) ;
#4125=EDGE_CURVE ( 'NONE', #6512, #13055, #3881, .T. ) ;
#4128=EDGE_LOOP ( 'NONE', ( #2997, #7767, #13560, #260 ) ) ;
#4133=EDGE_LOOP ( 'NONE', ( #7632, #3269, #2083, #5272, #10715, #5606 ) ) ;
#4134=CARTESIAN_POINT ( 'NONE',  ( -15.49969986081099904, -57.00737899243800655, 19.50231026484399877 ) ) ;
#4149=ORIENTED_EDGE ( 'NONE', *, *, #6043, .F. ) ;
#4169=CARTESIAN_POINT ( 'NONE',  ( -11.95473997639952302, -37.33086289605605401, 56.83510453573490651 ) ) ;
#4191=CARTESIAN_POINT ( 'NONE',  ( -7.660032944547833011, -48.43376236753700681, 21.09577438474947186 ) ) ;
#4197=( BOUNDED_CURVE ( )  B_SPLINE_CURVE ( 3, ( #7725, #3380, #12568, #12410 ),
 .UNSPECIFIED., .F., .F. ) 
 B_SPLINE_CURVE_WITH_KNOTS ( ( 4, 4 ),
 ( 5.060245233341797544, 5.259239931080632147 ),
 .UNSPECIFIED. ) 
 CURVE ( )  GEOMETRIC_REPRESENTATION_ITEM ( )  RATIONAL_B_SPLINE_CURVE ( ( 1.000000000000000000, 0.9967028139718016044, 0.9967028139718016044, 1.000000000000000000 ) ) 
 REPRESENTATION_ITEM ( '' )  );
#4203=EDGE_CURVE ( 'NONE', #7811, #1260, #7221, .T. ) ;
#4208=FACE_OUTER_BOUND ( 'NONE', #5751, .T. ) ;
#4209=CARTESIAN_POINT ( 'NONE',  ( -8.660471612933879015, -48.65904406005358851, 45.78551480191092793 ) ) ;
#4216=CYLINDRICAL_SURFACE ( 'NONE', #8941, 2.999999999999999112 ) ;
#4222=DIRECTION ( 'NONE',  ( 0.000000000000000000, 0.000000000000000000, -1.000000000000000000 ) ) ;
#4232=EDGE_CURVE ( 'NONE', #10290, #2754, #14094, .T. ) ;
#4242=CARTESIAN_POINT ( 'NONE',  ( -15.49969986081099194, -27.00737899243800300, 11.50231026484399877 ) ) ;
#4254=DIRECTION ( 'NONE',  ( -1.054621095516909827E-16, 0.000000000000000000, 1.000000000000000000 ) ) ;
#4260=FACE_BOUND ( 'NONE', #5550, .T. ) ;
#4262=ORIENTED_EDGE ( 'NONE', *, *, #3311, .T. ) ;
#4281=CARTESIAN_POINT ( 'NONE',  ( -8.010324353647195750, -47.33175634226493855, 56.24696452326014651 ) ) ;
#4286=( BOUNDED_CURVE ( )  B_SPLINE_CURVE ( 3, ( #5782, #4570, #3276, #5852 ),
 .UNSPECIFIED., .F., .F. ) 
 B_SPLINE_CURVE_WITH_KNOTS ( ( 4, 4 ),
 ( 5.038118467679318258, 5.213043692789276484 ),
 .UNSPECIFIED. ) 
 CURVE ( )  GEOMETRIC_REPRESENTATION_ITEM ( )  RATIONAL_B_SPLINE_CURVE ( ( 1.000000000000000000, 0.9974517222217440526, 0.9974517222217440526, 1.000000000000000000 ) ) 
 REPRESENTATION_ITEM ( '' )  );
#4287=CARTESIAN_POINT ( 'NONE',  ( -15.57469986081333424, -23.50709773848279482, 57.00223526477140013 ) ) ;
#4289=PLANE ( 'NONE',  #5927 ) ;
#4297=APPLICATION_CONTEXT ( 'automotive_design' ) ;
#4301=ORIENTED_EDGE ( 'NONE', *, *, #12681, .T. ) ;
#4302=VECTOR ( 'NONE', #1669, 1000.000000000000000 ) ;
#4308=VECTOR ( 'NONE', #2749, 1000.000000000000000 ) ;
#4311=LINE ( 'NONE', #5601, #12162 ) ;
#4320=CARTESIAN_POINT ( 'NONE',  ( -7.757642952717569429, -42.42537882359017942, 56.19456526637834770 ) ) ;
#4321=AXIS2_PLACEMENT_3D ( 'NONE', #768, #13697, #3137 ) ;
#4340=DIRECTION ( 'NONE',  ( 0.000000000000000000, -1.000000000000000000, -1.224646799147350002E-16 ) ) ;
#4357=VERTEX_POINT ( 'NONE', #13047 ) ;
#4364=LINE ( 'NONE', #3134, #4708 ) ;
#4381=CARTESIAN_POINT ( 'NONE',  ( 0.000000000000000000, 0.000000000000000000, 0.000000000000000000 ) ) ;
#4386=CARTESIAN_POINT ( 'NONE',  ( -7.886584594865190034, -46.96511696614950182, -7.955427708867500058 ) ) ;
#4402=EDGE_CURVE ( 'NONE', #5287, #11156, #13344, .T. ) ;
#4410=DIRECTION ( 'NONE',  ( 0.000000000000000000, -1.000000000000000000, -1.224646799147350002E-16 ) ) ;
#4413=CARTESIAN_POINT ( 'NONE',  ( -23.49969986081099904, -19.50737899243800300, 56.13904046828879757 ) ) ;
#4415=CARTESIAN_POINT ( 'NONE',  ( -18.32592690080561937, -37.01861151523911531, -17.89183167732498347 ) ) ;
#4431=ORIENTED_EDGE ( 'NONE', *, *, #10567, .T. ) ;
#4453=DIRECTION ( 'NONE',  ( 0.000000000000000000, 0.000000000000000000, -1.000000000000000000 ) ) ;
#4460=AXIS2_PLACEMENT_3D ( 'NONE', #2045, #4491, #1970 ) ;
#4477=CARTESIAN_POINT ( 'NONE',  ( -7.510659772263728051, -44.94657923994442683, 21.45543621087858810 ) ) ;
#4485=AXIS2_PLACEMENT_3D ( 'NONE', #1751, #10007, #5346 ) ;
#4487=CARTESIAN_POINT ( 'NONE',  ( -16.02889839021359819, -36.52059104800384404, -17.99486483221301114 ) ) ;
#4491=DIRECTION ( 'NONE',  ( 0.000000000000000000, -1.000000000000000000, -1.224646799147350002E-16 ) ) ;
#4495=CARTESIAN_POINT ( 'NONE',  ( 7.500300139189000070, -37.00737899243799944, -10.11609617439569675 ) ) ;
#4504=FACE_OUTER_BOUND ( 'NONE', #9754, .T. ) ;
#4512=ADVANCED_FACE ( 'NONE', ( #12490 ), #4532, .F. ) ;
#4513=EDGE_CURVE ( 'NONE', #3128, #14077, #7728, .T. ) ;
#4514=ADVANCED_FACE ( 'NONE', ( #6577 ), #5592, .F. ) ;
#4516=CARTESIAN_POINT ( 'NONE',  ( -8.835531075157819103, -48.93602667744891477, 45.18199390436557650 ) ) ;
#4517=( BOUNDED_CURVE ( )  B_SPLINE_CURVE ( 3, ( #4110, #13308, #8546, #4038 ),
 .UNSPECIFIED., .F., .F. ) 
 B_SPLINE_CURVE_WITH_KNOTS ( ( 4, 4 ),
 ( 3.141592653589793560, 4.400121501412660230 ),
 .UNSPECIFIED. ) 
 CURVE ( )  GEOMETRIC_REPRESENTATION_ITEM ( )  RATIONAL_B_SPLINE_CURVE ( ( 1.000000000000000000, 0.8723071003127499390, 0.8723071003127499390, 1.000000000000000000 ) ) 
 REPRESENTATION_ITEM ( '' )  );
#4523=DIRECTION ( 'NONE',  ( 0.000000000000000000, 0.000000000000000000, -1.000000000000000000 ) ) ;
#4529=ORIENTED_EDGE ( 'NONE', *, *, #1798, .T. ) ;
#4532=PLANE ( 'NONE',  #6810 ) ;
#4535=VERTEX_POINT ( 'NONE', #4608 ) ;
#4537=CARTESIAN_POINT ( 'NONE',  ( -19.04823043207872502, -51.68209199896817552, -17.83013874036776514 ) ) ;
#4540=ORIENTED_EDGE ( 'NONE', *, *, #3060, .T. ) ;
#4542=DIRECTION ( 'NONE',  ( -3.632077277826439854E-16, 1.000000000000000000, 0.000000000000000000 ) ) ;
#4553=CARTESIAN_POINT ( 'NONE',  ( -34.99969986081099904, -20.37340439622244048, -12.21913358627979918 ) ) ;
#4561=CARTESIAN_POINT ( 'NONE',  ( -23.49969986081100259, -44.50737899243799944, -17.13441993860073254 ) ) ;
#4570=CARTESIAN_POINT ( 'NONE',  ( -29.57393575939414632, -54.93314309385485217, -15.32525311590548966 ) ) ;
#4576=DIRECTION ( 'NONE',  ( 1.000000000000000000, -1.291538348938060198E-32, 1.054621095516909827E-16 ) ) ;
#4580=EDGE_LOOP ( 'NONE', ( #95, #7669, #2167, #6083 ) ) ;
#4581=FACE_OUTER_BOUND ( 'NONE', #10267, .T. ) ;
#4585=VECTOR ( 'NONE', #6623, 1000.000000000000000 ) ;
#4592=EDGE_CURVE ( 'NONE', #10639, #1735, #14648, .T. ) ;
#4607=( BOUNDED_CURVE ( )  B_SPLINE_CURVE ( 3, ( #13210, #2714, #7367, #12053 ),
 .UNSPECIFIED., .F., .F. ) 
 B_SPLINE_CURVE_WITH_KNOTS ( ( 4, 4 ),
 ( 1.570796326794895004, 3.141592653589793560 ),
 .UNSPECIFIED. ) 
 CURVE ( )  GEOMETRIC_REPRESENTATION_ITEM ( )  RATIONAL_B_SPLINE_CURVE ( ( 1.000000000000000000, 0.8047378541243644934, 0.8047378541243644934, 1.000000000000000000 ) ) 
 REPRESENTATION_ITEM ( '' )  );
#4608=CARTESIAN_POINT ( 'NONE',  ( 4.000300139189000959, -19.50737899243798879, 51.53354502093799994 ) ) ;
#4610=FACE_OUTER_BOUND ( 'NONE', #2522, .T. ) ;
#4615=CARTESIAN_POINT ( 'NONE',  ( 6.912059853347208183, -37.03279448458209089, -10.56576583290206806 ) ) ;
#4621=CARTESIAN_POINT ( 'NONE',  ( -20.31756358285883479, -22.27118552192390055, 56.69196217374378222 ) ) ;
#4623=VECTOR ( 'NONE', #13558, 1000.000000000000000 ) ;
#4627=PLANE ( 'NONE',  #11601 ) ;
#4629=VECTOR ( 'NONE', #8788, 1000.000000000000000 ) ;
#4630=CARTESIAN_POINT ( 'NONE',  ( -7.512043759983883184, -44.96869557946827456, 21.47290527092978607 ) ) ;
#4632=DIRECTION ( 'NONE',  ( 0.000000000000000000, 0.000000000000000000, 1.000000000000000000 ) ) ;
#4634=CARTESIAN_POINT ( 'NONE',  ( -7.705200311943016800, -46.31941204765107045, 42.00231026484399166 ) ) ;
#4645=ADVANCED_FACE ( 'NONE', ( #3530 ), #2537, .F. ) ;
#4648=LINE ( 'NONE', #9302, #5797 ) ;
#4659=LINE ( 'NONE', #6015, #11534 ) ;
#4668=CARTESIAN_POINT ( 'NONE',  ( -7.773685182324116205, -47.89679818372221831, -7.581023005281736005 ) ) ;
#4672=CARTESIAN_POINT ( 'NONE',  ( -5.499699860810998153, -46.50737899243799944, -2.497689735156003010 ) ) ;
#4691=CARTESIAN_POINT ( 'NONE',  ( -16.02307658328272311, -52.50737899243798523, -17.99768973515599413 ) ) ;
#4694=CARTESIAN_POINT ( 'NONE',  ( 3.284438305224395283, -39.31204358972114932, -12.95406313883616356 ) ) ;
#4699=CARTESIAN_POINT ( 'NONE',  ( 4.095996200104924156, -38.34531428877323123, 51.47509614191934446 ) ) ;
#4703=CARTESIAN_POINT ( 'NONE',  ( -11.02342383152547356, -36.50737899243797102, -13.49768973515603321 ) ) ;
#4707=VECTOR ( 'NONE', #9699, 1000.000000000000000 ) ;
#4708=VECTOR ( 'NONE', #8939, 1000.000000000000000 ) ;
#4709=CARTESIAN_POINT ( 'NONE',  ( -7.504323356601999784, -44.76276341930999081, 21.29631823119984091 ) ) ;
#4712=ORIENTED_EDGE ( 'NONE', *, *, #2386, .F. ) ;
#4713=CYLINDRICAL_SURFACE ( 'NONE', #6041, 8.000000000000000000 ) ;
#4714=DIRECTION ( 'NONE',  ( 0.000000000000000000, 1.224646799147350002E-16, -1.000000000000000000 ) ) ;
#4716=ORIENTED_EDGE ( 'NONE', *, *, #6896, .T. ) ;
#4718=CARTESIAN_POINT ( 'NONE',  ( -5.499699860810998153, -46.50737899243799944, -5.497689735156003010 ) ) ;
#4721=CARTESIAN_POINT ( 'NONE',  ( -14.97186396627019533, -36.50737899243800655, -17.99768973515599768 ) ) ;
#4723=AXIS2_PLACEMENT_3D ( 'NONE', #12176, #8573, #11101 ) ;
#4727=CARTESIAN_POINT ( 'NONE',  ( -20.18599136182623965, -36.50737899243796392, -13.49768973515603498 ) ) ;
#4752=DIRECTION ( 'NONE',  ( 1.000000000000000000, -1.291538348938060198E-32, 1.054621095516909827E-16 ) ) ;
#4754=EDGE_LOOP ( 'NONE', ( #6982, #14620, #11516, #3996, #5037, #299, #8579, #2191, #11800, #6654, #5308, #11086 ) ) ;
#4769=CARTESIAN_POINT ( 'NONE',  ( 2.819042285013538596, -40.24211141612355647, -13.21890428332254963 ) ) ;
#4773=ORIENTED_EDGE ( 'NONE', *, *, #9247, .T. ) ;
#4777=ORIENTED_EDGE ( 'NONE', *, *, #9257, .T. ) ;
#4780=FACE_OUTER_BOUND ( 'NONE', #9505, .T. ) ;
#4785=CARTESIAN_POINT ( 'NONE',  ( -7.658052939403637183, -48.44202655475368857, -3.914257181409824593 ) ) ;
#4794=CARTESIAN_POINT ( 'NONE',  ( -23.35746721609777055, -42.93911546747612107, 56.16991628440959516 ) ) ;
#4806=VERTEX_POINT ( 'NONE', #9658 ) ;
#4809=CARTESIAN_POINT ( 'NONE',  ( -7.508316264967583642, -44.14096455381468331, -6.326192033447865626 ) ) ;
#4816=VECTOR ( 'NONE', #13773, 1000.000000000000000 ) ;
#4819=EDGE_CURVE ( 'NONE', #569, #2126, #11025, .T. ) ;
#4824=CARTESIAN_POINT ( 'NONE',  ( -12.67520354219633383, -51.99671047118290090, -17.89194748959578263 ) ) ;
#4828=ORIENTED_EDGE ( 'NONE', *, *, #2804, .T. ) ;
#4846=CARTESIAN_POINT ( 'NONE',  ( 3.032897922443514638, -39.75996117776323047, -13.09822540226690357 ) ) ;
#4848=CARTESIAN_POINT ( 'NONE',  ( -15.49969986081099371, -57.00737899243799944, -17.99768973515599768 ) ) ;
#4849=EDGE_LOOP ( 'NONE', ( #5744, #7078, #11085, #12852, #4034, #1311 ) ) ;
#4852=B_SPLINE_CURVE_WITH_KNOTS ( 'NONE', 3,
 ( #2969, #6475, #1904, #9928, #7628, #13535, #12384, #11158, #677, #12539, #5344, #5562, #13610, #13758, #2056, #9005, #11310, #13685, #8855, #7845, #5492, #11383, #6403 ),
 .UNSPECIFIED., .F., .F.,
 ( 4, 2, 2, 2, 2, 2, 2, 2, 1, 1, 1, 2, 4 ),
 ( 0.1213360741398818166, 0.1630074590234368292, 0.2046788439069918142, 0.2880216136741018396, 0.4547071532083220013, 0.5380499229754320822, 0.5588856154172106017, 0.5614900769724329166, 0.5640945385276554536, 0.5693034616381122959, 0.5797213078590257584, 0.6213926927426793867, 0.7880782322772789117 ),
 .UNSPECIFIED. ) ;
#4857=EDGE_CURVE ( 'NONE', #7229, #5221, #1071, .T. ) ;
#4864=CARTESIAN_POINT ( 'NONE',  ( -7.506424547597141839, -48.98717474752383083, -5.822033054479117453 ) ) ;
#4869=ORIENTED_EDGE ( 'NONE', *, *, #12574, .F. ) ;
#4872=CARTESIAN_POINT ( 'NONE',  ( -15.49969986081099904, -36.50737899243799944, 57.00231026484399877 ) ) ;
#4873=ORIENTED_EDGE ( 'NONE', *, *, #7572, .F. ) ;
#4879=EDGE_CURVE ( 'NONE', #4535, #9803, #10021, .T. ) ;
#4888=ORIENTED_EDGE ( 'NONE', *, *, #9757, .F. ) ;
#4908=ORIENTED_EDGE ( 'NONE', *, *, #12103, .T. ) ;
#4909=CARTESIAN_POINT ( 'NONE',  ( -33.50952539253209039, -41.64595657058005429, -13.38988768305012123 ) ) ;
#4912=EDGE_CURVE ( 'NONE', #3278, #6631, #1208, .T. ) ;
#4913=CIRCLE ( 'NONE', #3435, 37.50000000000000000 ) ;
#4921=CARTESIAN_POINT ( 'NONE',  ( 2.734184828063399575, -40.49459960338367637, -13.26621881384550861 ) ) ;
#4935=CARTESIAN_POINT ( 'NONE',  ( -7.660032944547864986, -48.43376236753701392, -3.904225615250556114 ) ) ;
#4937=ORIENTED_EDGE ( 'NONE', *, *, #38, .F. ) ;
#4941=VERTEX_POINT ( 'NONE', #8269 ) ;
#4944=CARTESIAN_POINT ( 'NONE',  ( -16.02267528388033213, -36.50737899243799944, 57.00231026484399877 ) ) ;
#4945=EDGE_LOOP ( 'NONE', ( #12799, #6285, #12300, #4873, #3617, #6958 ) ) ;
#4992=AXIS2_PLACEMENT_3D ( 'NONE', #3097, #13363, #6455 ) ;
#5010=DIRECTION ( 'NONE',  ( 0.000000000000000000, -1.000000000000000000, -1.224646799147350002E-16 ) ) ;
#5013=DIRECTION ( 'NONE',  ( 0.000000000000000000, 0.000000000000000000, 1.000000000000000000 ) ) ;
#5018=CARTESIAN_POINT ( 'NONE',  ( 2.500300139188999626, -46.50737899243799944, -7.997689735156003010 ) ) ;
#5022=PLANE ( 'NONE',  #9321 ) ;
#5027=CARTESIAN_POINT ( 'NONE',  ( -9.226714359780459063, -21.29551127497027707, 56.47371171714189586 ) ) ;
#5035=DIRECTION ( 'NONE',  ( 0.000000000000000000, -1.000000000000000000, -1.224646799147350002E-16 ) ) ;
#5037=ORIENTED_EDGE ( 'NONE', *, *, #2614, .F. ) ;
#5041=LINE ( 'NONE', #5113, #4707 ) ;
#5044=CARTESIAN_POINT ( 'NONE',  ( -7.516520390631877824, -48.95538363176652297, 18.97731922801482440 ) ) ;
#5045=ADVANCED_FACE ( 'NONE', ( #8467 ), #379, .F. ) ;
#5048=EDGE_CURVE ( 'NONE', #5628, #7811, #10617, .T. ) ;
#5050=CARTESIAN_POINT ( 'NONE',  ( -7.768786321151917917, -46.58155647109239084, -17.19222724300273342 ) ) ;
#5055=CARTESIAN_POINT ( 'NONE',  ( -33.49969986081099904, -51.00737899243799944, -13.39525803434800011 ) ) ;
#5070=LINE ( 'NONE', #12329, #3963 ) ;
#5094=ORIENTED_EDGE ( 'NONE', *, *, #4402, .T. ) ;
#5110=ORIENTED_EDGE ( 'NONE', *, *, #12681, .F. ) ;
#5111=CARTESIAN_POINT ( 'NONE',  ( -5.499699860810997265, -46.50737899243799944, -5.497689735156003010 ) ) ;
#5113=CARTESIAN_POINT ( 'NONE',  ( -7.499699860810999041, -44.50737899243799944, -109.5506571639849938 ) ) ;
#5117=CARTESIAN_POINT ( 'NONE',  ( -7.752363797594753692, -48.01475789269077410, 17.50266728317557963 ) ) ;
#5121=CARTESIAN_POINT ( 'NONE',  ( -7.705135643603000517, -46.32754971434033564, -17.17871339279434295 ) ) ;
#5126=CARTESIAN_POINT ( 'NONE',  ( -7.754796638793765240, -46.50763592918296752, 17.00313569000094560 ) ) ;
#5131=CARTESIAN_POINT ( 'NONE',  ( -5.499699860810998153, -46.50737899243799944, -8.497689735156003010 ) ) ;
#5133=EDGE_CURVE ( 'NONE', #6753, #7373, #957, .T. ) ;
#5137=CARTESIAN_POINT ( 'NONE',  ( -7.500924733540946576, -44.35427680771954329, 45.77981586235881650 ) ) ;
#5146=ORIENTED_EDGE ( 'NONE', *, *, #10557, .T. ) ;
#5153=CARTESIAN_POINT ( 'NONE',  ( 2.500300139189002291, -46.50737899243799944, -8.497689735156001234 ) ) ;
#5161=ORIENTED_EDGE ( 'NONE', *, *, #8209, .F. ) ;
#5162=LINE ( 'NONE', #8749, #9338 ) ;
#5163=ADVANCED_FACE ( 'NONE', ( #9773, #4260 ), #12371, .T. ) ;
#5171=EDGE_LOOP ( 'NONE', ( #13803, #318 ) ) ;
#5172=CARTESIAN_POINT ( 'NONE',  ( -15.49969986081099194, -27.00737899243800300, 19.50231026484399877 ) ) ;
#5178=CARTESIAN_POINT ( 'NONE',  ( -33.49969986081099904, -51.00737899243799944, 52.39987856403599409 ) ) ;
#5182=AXIS2_PLACEMENT_3D ( 'NONE', #5277, #8715, #10085 ) ;
#5184=CARTESIAN_POINT ( 'NONE',  ( -7.886584594865180264, -46.96511696614940234, -3.039951761444701361 ) ) ;
#5194=CARTESIAN_POINT ( 'NONE',  ( -15.57469986081099478, -26.50737899243800300, 56.85231026484400019 ) ) ;
#5197=CARTESIAN_POINT ( 'NONE',  ( -34.85309570014907621, -38.58518656690294790, -12.61778470598987312 ) ) ;
#5198=EDGE_LOOP ( 'NONE', ( #7273, #5915 ) ) ;
#5207=CARTESIAN_POINT ( 'NONE',  ( -15.49969986081099904, -13.50737899243800122, 56.85231026484400019 ) ) ;
#5218=CARTESIAN_POINT ( 'NONE',  ( -3.499699860810999041, -57.00737899243800655, 55.03046811182510112 ) ) ;
#5219=CARTESIAN_POINT ( 'NONE',  ( -7.498763094504910853, -44.75646166653845626, -7.292659265823624004 ) ) ;
#5221=VERTEX_POINT ( 'NONE', #13597 ) ;
#5226=DIRECTION ( 'NONE',  ( 1.000000000000000000, 0.000000000000000000, 0.000000000000000000 ) ) ;
#5233=EDGE_CURVE ( 'NONE', #11156, #2347, #10058, .T. ) ;
#5235=LINE ( 'NONE', #427, #8978 ) ;
#5241=CARTESIAN_POINT ( 'NONE',  ( -23.49969986081100970, -45.03523210613074212, 56.13904046828874073 ) ) ;
#5244=CARTESIAN_POINT ( 'NONE',  ( -14.18877560904499902, -36.61116194625252973, 56.98027335662509074 ) ) ;
#5247=AXIS2_PLACEMENT_3D ( 'NONE', #767, #846, #10013 ) ;
#5248=CARTESIAN_POINT ( 'NONE',  ( -9.119211481053252299, -21.20735069469006717, 56.45528369196469498 ) ) ;
#5251=CARTESIAN_POINT ( 'NONE',  ( -5.499699860811000818, -46.50737899243799944, 19.50231026484399877 ) ) ;
#5271=B_SPLINE_CURVE_WITH_KNOTS ( 'NONE', 3,
 ( #2263, #8058, #15106, #12749, #5543, #11591, #1108, #5766, #4634, #2034 ),
 .UNSPECIFIED., .F., .F.,
 ( 4, 2, 2, 2, 4 ),
 ( 0.005531701047751949943, 0.006113612598919536401, 0.006695524150087122858, 0.007277435701254709316, 0.007859347252422295774 ),
 .UNSPECIFIED. ) ;
#5272=ORIENTED_EDGE ( 'NONE', *, *, #11015, .T. ) ;
#5274=DIRECTION ( 'NONE',  ( 0.000000000000000000, 0.000000000000000000, 1.000000000000000000 ) ) ;
#5276=EDGE_CURVE ( 'NONE', #11014, #5496, #5477, .T. ) ;
#5277=CARTESIAN_POINT ( 'NONE',  ( -15.49969986081099194, -32.00737899243799944, 19.50231026484399166 ) ) ;
#5283=DIRECTION ( 'NONE',  ( 0.000000000000000000, 1.000000000000000000, 1.224646799147350002E-16 ) ) ;
#5284=CARTESIAN_POINT ( 'NONE',  ( -7.499699860810999930, -44.42675748898079036, 45.89481492690103437 ) ) ;
#5287=VERTEX_POINT ( 'NONE', #10217 ) ;
#5290=ORIENTED_EDGE ( 'NONE', *, *, #5870, .T. ) ;
#5292=CARTESIAN_POINT ( 'NONE',  ( -15.49969986081099904, -57.00737899243800655, 19.50231026484399877 ) ) ;
#5297=EDGE_CURVE ( 'NONE', #12356, #777, #11903, .T. ) ;
#5308=ORIENTED_EDGE ( 'NONE', *, *, #10557, .F. ) ;
#5309=ORIENTED_EDGE ( 'NONE', *, *, #14539, .T. ) ;
#5313=CARTESIAN_POINT ( 'NONE',  ( -12.19373306175957161, -37.21772783548635744, 56.85708728699461290 ) ) ;
#5320=CIRCLE ( 'NONE', #1418, 3.000000000000002665 ) ;
#5323=CARTESIAN_POINT ( 'NONE',  ( 2.500300139188999182, -46.50737899243799944, 44.50231026484399877 ) ) ;
#5326=DIRECTION ( 'NONE',  ( 0.000000000000000000, -1.000000000000000000, -1.224646799147350002E-16 ) ) ;
#5331=CARTESIAN_POINT ( 'NONE',  ( -27.49969986081100259, -57.00737899243800655, 55.03046811182510112 ) ) ;
#5334=EDGE_CURVE ( 'NONE', #9659, #6512, #14635, .T. ) ;
#5335=EDGE_CURVE ( 'NONE', #11647, #2093, #3473, .T. ) ;
#5344=CARTESIAN_POINT ( 'NONE',  ( -7.519587752637010070, -45.08058686818623784, -3.441745684778983794 ) ) ;
#5346=DIRECTION ( 'NONE',  ( -1.734723475976807094E-16, 0.000000000000000000, 1.000000000000000000 ) ) ;
#5356=FACE_OUTER_BOUND ( 'NONE', #10252, .T. ) ;
#5366=CARTESIAN_POINT ( 'NONE',  ( -7.532278898138853762, -45.22326128447397764, -7.645014517789088693 ) ) ;
#5369=PLANE ( 'NONE',  #5557 ) ;
#5371=ORIENTED_EDGE ( 'NONE', *, *, #8966, .T. ) ;
#5373=FACE_OUTER_BOUND ( 'NONE', #13216, .T. ) ;
#5376=CARTESIAN_POINT ( 'NONE',  ( 2.500300139188999182, -46.50737899243799944, 19.50231026484399877 ) ) ;
#5377=EDGE_CURVE ( 'NONE', #11014, #8446, #9449, .T. ) ;
#5380=FACE_OUTER_BOUND ( 'NONE', #3100, .T. ) ;
#5385=FACE_OUTER_BOUND ( 'NONE', #4754, .T. ) ;
#5393=DIRECTION ( 'NONE',  ( 0.000000000000000000, 0.000000000000000000, -1.000000000000000000 ) ) ;
#5405=DIRECTION ( 'NONE',  ( 1.000000000000000000, -1.291538348938060198E-32, 1.054621095516909827E-16 ) ) ;
#5411=ORIENTED_EDGE ( 'NONE', *, *, #4857, .T. ) ;
#5412=CARTESIAN_POINT ( 'NONE',  ( -28.28282149594069850, -32.00737899243799944, 54.75627176226269199 ) ) ;
#5416=ORIENTED_EDGE ( 'NONE', *, *, #5133, .F. ) ;
#5417=CARTESIAN_POINT ( 'NONE',  ( -7.512805849530849400, -44.04964101872660365, -5.039951761444699585 ) ) ;
#5421=CARTESIAN_POINT ( 'NONE',  ( -14.44815700838962691, -52.45516431684754366, 56.99107276615496431 ) ) ;
#5422=ADVANCED_FACE ( 'NONE', ( #11981, #51 ), #5022, .T. ) ;
#5425=CARTESIAN_POINT ( 'NONE',  ( -8.185742736628769833, -47.75198331066174262, 46.67630207578714163 ) ) ;
#5426=VECTOR ( 'NONE', #2512, 1000.000000000000000 ) ;
#5428=FACE_OUTER_BOUND ( 'NONE', #3936, .T. ) ;
#5439=CARTESIAN_POINT ( 'NONE',  ( -7.838472470387507940, -46.81608433807591751, 17.01681591762138979 ) ) ;
#5445=EDGE_CURVE ( 'NONE', #12587, #9659, #2579, .T. ) ;
#5454=DIRECTION ( 'NONE',  ( 1.000000000000000000, -1.291538348938060198E-32, 1.054621095516909827E-16 ) ) ;
#5455=EDGE_LOOP ( 'NONE', ( #8237, #6647, #13760, #9122 ) ) ;
#5456=EDGE_LOOP ( 'NONE', ( #10483, #5094, #2062, #7611, #297 ) ) ;
#5459=ORIENTED_EDGE ( 'NONE', *, *, #8796, .F. ) ;
#5477=LINE ( 'NONE', #1045, #7128 ) ;
#5478=CARTESIAN_POINT ( 'NONE',  ( -7.886584594865190034, -46.96511696614940234, 17.04457229113261718 ) ) ;
#5492=CARTESIAN_POINT ( 'NONE',  ( -7.504307622470381745, -44.76319932751670194, -3.703265526006389141 ) ) ;
#5494=ORIENTED_EDGE ( 'NONE', *, *, #9875, .F. ) ;
#5495=CARTESIAN_POINT ( 'NONE',  ( -15.49969986081099904, -26.50737899243800300, 19.50231026484400232 ) ) ;
#5496=VERTEX_POINT ( 'NONE', #11050 ) ;
#5522=VERTEX_POINT ( 'NONE', #4088 ) ;
#5523=LINE ( 'NONE', #10033, #7356 ) ;
#5525=EDGE_LOOP ( 'NONE', ( #1001, #13283, #7508, #7652, #6573 ) ) ;
#5530=VERTEX_POINT ( 'NONE', #14646 ) ;
#5532=ORIENTED_EDGE ( 'NONE', *, *, #3966, .T. ) ;
#5533=CARTESIAN_POINT ( 'NONE',  ( -9.658903420740534429, -39.03434883555972590, 56.54512877198791898 ) ) ;
#5537=AXIS2_PLACEMENT_3D ( 'NONE', #11498, #7891, #12582 ) ;
#5543=CARTESIAN_POINT ( 'NONE',  ( -7.529819136880052888, -45.22287388988081602, 42.34868737210720724 ) ) ;
#5544=CIRCLE ( 'NONE', #7499, 8.000000000000000000 ) ;
#5550=EDGE_LOOP ( 'NONE', ( #12696, #15075 ) ) ;
#5551=FACE_OUTER_BOUND ( 'NONE', #10237, .T. ) ;
#5557=AXIS2_PLACEMENT_3D ( 'NONE', #13708, #15003, #935 ) ;
#5562=CARTESIAN_POINT ( 'NONE',  ( -7.512025533959445056, -44.96883993545320379, -3.526982330024790446 ) ) ;
#5569=CARTESIAN_POINT ( 'NONE',  ( -7.922155832732967973, -47.08606123773714813, 56.22882524374293212 ) ) ;
#5571=CARTESIAN_POINT ( 'NONE',  ( -8.551496829098008234, -48.47395512894357950, 42.95037523886164621 ) ) ;
#5573=VECTOR ( 'NONE', #10893, 1000.000000000000000 ) ;
#5588=EDGE_CURVE ( 'NONE', #13722, #8988, #6133, .T. ) ;
#5592=PLANE ( 'NONE',  #8771 ) ;
#5593=B_SPLINE_CURVE_WITH_KNOTS ( 'NONE', 3,
 ( #2300, #11621, #5805, #2450, #163, #11855, #9, #9325, #10325, #8175, #12862, #2377, #9483, #7016, #11698, #1223, #13020, #14155, #14993, #5874, #3899, #14452, #3819, #13090, #7245, #2826, #12157, #10708, #1599, #14232, #9556, #9637, #2753, #12089, #7480, #11935 ),
 .UNSPECIFIED., .F., .F.,
 ( 4, 2, 1, 1, 1, 2, 2, 2, 1, 1, 1, 2, 2, 2, 2, 2, 2, 2, 2, 2, 4 ),
 ( 0.000000000000000000, 0.1249999999999846789, 0.1874999999999764910, 0.2187499999999724110, 0.2343749999999710232, 0.2421874999999706624, 0.2499999999999703015, 0.3749999999999719669, 0.4374999999999742983, 0.4687499999999745759, 0.4843749999999745204, 0.4921874999999732991, 0.4999999999999720224, 0.6249999999999749090, 0.6874999999999754641, 0.7187499999999766853, 0.7499999999999780176, 0.8124999999999826805, 0.8437499999999856781, 0.8749999999999887867, 1.000000000000000000 ),
 .UNSPECIFIED. ) ;
#5596=CIRCLE ( 'NONE', #8536, 3.000000000000002665 ) ;
#5600=EDGE_LOOP ( 'NONE', ( #13286, #12388 ) ) ;
#5601=CARTESIAN_POINT ( 'NONE',  ( -2.716578225681299141, -32.00737899243799944, -17.99768973515599768 ) ) ;
#5606=ORIENTED_EDGE ( 'NONE', *, *, #4087, .F. ) ;
#5607=CARTESIAN_POINT ( 'NONE',  ( 2.788504248039533451, -40.33206847769235992, 52.24055437141020519 ) ) ;
#5611=CARTESIAN_POINT ( 'NONE',  ( -15.49969986081099904, -13.50737899243800122, 54.00231026484400587 ) ) ;
#5613=CARTESIAN_POINT ( 'NONE',  ( -7.660976687611689151, -46.08634367607207594, 21.96889143210171014 ) ) ;
#5620=FACE_OUTER_BOUND ( 'NONE', #9900, .T. ) ;
#5623=CARTESIAN_POINT ( 'NONE',  ( -15.49969986081099904, -27.00737899243800300, -5.497689735156002122 ) ) ;
#5625=AXIS2_PLACEMENT_3D ( 'NONE', #174, #5972, #2613 ) ;
#5626=CARTESIAN_POINT ( 'NONE',  ( -20.37940433654428318, -38.14658552601336083, -17.68140352835245110 ) ) ;
#5628=VERTEX_POINT ( 'NONE', #7813 ) ;
#5633=CARTESIAN_POINT ( 'NONE',  ( -7.658052939403637183, -48.44202655475336172, 21.08574281859059241 ) ) ;
#5648=CARTESIAN_POINT ( 'NONE',  ( -8.370866812342363517, -48.14008301383953636, 42.60233345630671664 ) ) ;
#5665=( BOUNDED_CURVE ( )  B_SPLINE_CURVE ( 3, ( #7852, #12548, #9088, #12623 ),
 .UNSPECIFIED., .F., .T. ) 
 B_SPLINE_CURVE_WITH_KNOTS ( ( 4, 4 ),
 ( 1.023945376098953863, 1.222940073837788688 ),
 .UNSPECIFIED. ) 
 CURVE ( )  GEOMETRIC_REPRESENTATION_ITEM ( )  RATIONAL_B_SPLINE_CURVE ( ( 1.000000000000000000, 0.9967028139718016044, 0.9967028139718016044, 1.000000000000000000 ) ) 
 REPRESENTATION_ITEM ( '' )  );
#5675=DIRECTION ( 'NONE',  ( 0.000000000000000000, -1.000000000000000000, -1.224646799147350002E-16 ) ) ;
#5678=VERTEX_POINT ( 'NONE', #4242 ) ;
#5690=EDGE_CURVE ( 'NONE', #2418, #9903, #14607, .T. ) ;
#5691=CARTESIAN_POINT ( 'NONE',  ( -7.640766570737479668, -45.98099911298281484, 21.94864471303565878 ) ) ;
#5701=CIRCLE ( 'NONE', #11090, 37.50000000000000711 ) ;
#5702=VECTOR ( 'NONE', #4030, 1000.000000000000000 ) ;
#5703=CARTESIAN_POINT ( 'NONE',  ( -22.43025610151164173, -40.50285774858512866, -17.35190600379631221 ) ) ;
#5712=CARTESIAN_POINT ( 'NONE',  ( -7.499699860810997265, -44.50737899243797813, 46.00231026484399877 ) ) ;
#5715=CARTESIAN_POINT ( 'NONE',  ( -5.499699860811000818, -46.50737899243799944, 22.00231026484399877 ) ) ;
#5717=DIRECTION ( 'NONE',  ( 0.000000000000000000, 0.000000000000000000, -1.000000000000000000 ) ) ;
#5724=CARTESIAN_POINT ( 'NONE',  ( -7.512805849530849400, -44.04964101872660365, 19.96004823855532706 ) ) ;
#5725=CARTESIAN_POINT ( 'NONE',  ( -5.499699860811000818, -46.50737899243799944, 19.50231026484399877 ) ) ;
#5737=LINE ( 'NONE', #13783, #11904 ) ;
#5744=ORIENTED_EDGE ( 'NONE', *, *, #8772, .F. ) ;
#5751=EDGE_LOOP ( 'NONE', ( #3794, #6333 ) ) ;
#5760=CARTESIAN_POINT ( 'NONE',  ( -9.150909411738691546, -39.63286124672721655, 56.46135555955575569 ) ) ;
#5766=CARTESIAN_POINT ( 'NONE',  ( -7.663084634444070176, -46.12710533971196014, 42.02396812144193916 ) ) ;
#5770=CYLINDRICAL_SURFACE ( 'NONE', #5910, 8.000000000000000000 ) ;
#5772=CARTESIAN_POINT ( 'NONE',  ( -23.24232539787402274, -42.42616270815122448, -17.18982661429730641 ) ) ;
#5782=CARTESIAN_POINT ( 'NONE',  ( -27.49969986081100259, -57.00737899243800655, -16.02584758213710003 ) ) ;
#5792=CARTESIAN_POINT ( 'NONE',  ( -7.499699860810997265, -44.50737899243797813, 46.00231026484399877 ) ) ;
#5797=VECTOR ( 'NONE', #8154, 1000.000000000000000 ) ;
#5804=CIRCLE ( 'NONE', #7262, 37.50000000000000000 ) ;
#5805=CARTESIAN_POINT ( 'NONE',  ( -37.91145957496917163, -37.03279448458209799, 49.57038636259010644 ) ) ;
#5808=ORIENTED_EDGE ( 'NONE', *, *, #2915, .F. ) ;
#5813=ORIENTED_EDGE ( 'NONE', *, *, #10982, .F. ) ;
#5827=DIRECTION ( 'NONE',  ( -1.000000000000000000, -3.700743415417187646E-16, 0.000000000000000000 ) ) ;
#5836=CARTESIAN_POINT ( 'NONE',  ( -7.730209135540895282, -46.40248289166846973, 22.00066548116162224 ) ) ;
#5837=DIRECTION ( 'NONE',  ( 1.445602896647339656E-16, 0.000000000000000000, -1.000000000000000000 ) ) ;
#5846=CARTESIAN_POINT ( 'NONE',  ( -20.78589391471635039, -38.48009039869666736, 56.62973181049755311 ) ) ;
#5849=CARTESIAN_POINT ( 'NONE',  ( -15.49969986081099904, -37.00737899243799944, 19.50231026484399877 ) ) ;
#5851=CARTESIAN_POINT ( 'NONE',  ( -13.97717856230794631, -23.42060321925418265, 56.97738585718026627 ) ) ;
#5852=CARTESIAN_POINT ( 'NONE',  ( -33.49969986081099904, -51.00737899243799944, -13.39525803434800011 ) ) ;
#5854=EDGE_CURVE ( 'NONE', #569, #10290, #8835, .T. ) ;
#5862=CARTESIAN_POINT ( 'NONE',  ( -15.49969986081099371, -36.50737899243799944, -17.99768973515599768 ) ) ;
#5865=FACE_BOUND ( 'NONE', #5600, .T. ) ;
#5867=CARTESIAN_POINT ( 'NONE',  ( -8.005749619258239136, -47.31205335750601648, 46.87470529982511636 ) ) ;
#5870=EDGE_CURVE ( 'NONE', #13194, #4806, #7842, .T. ) ;
#5873=CARTESIAN_POINT ( 'NONE',  ( -7.671650320578205395, -48.38766871647334966, -7.145439208203410608 ) ) ;
#5874=CARTESIAN_POINT ( 'NONE',  ( -34.90864537991240724, -38.51142663665533661, 51.59020252618820024 ) ) ;
#5880=CARTESIAN_POINT ( 'NONE',  ( -5.499699860811003482, -46.50737899243799944, 41.50231026484399166 ) ) ;
#5882=EDGE_CURVE ( 'NONE', #6735, #2509, #1267, .T. ) ;
#5885=ORIENTED_EDGE ( 'NONE', *, *, #9474, .T. ) ;
#5889=FACE_OUTER_BOUND ( 'NONE', #48, .T. ) ;
#5902=CARTESIAN_POINT ( 'NONE',  ( 5.644331944133275769, -37.36437517128688057, 50.47299701629476942 ) ) ;
#5910=AXIS2_PLACEMENT_3D ( 'NONE', #5623, #11370, #8989 ) ;
#5913=CARTESIAN_POINT ( 'NONE',  ( -7.570456978157269035, -48.78587553030465784, -4.456442176039379532 ) ) ;
#5915=ORIENTED_EDGE ( 'NONE', *, *, #13423, .T. ) ;
#5921=CARTESIAN_POINT ( 'NONE',  ( -22.98851422383178544, -41.68127855727117748, 56.24708203345880975 ) ) ;
#5924=FILL_AREA_STYLE ('',( #1427 ) ) ;
#5927=AXIS2_PLACEMENT_3D ( 'NONE', #14920, #9098, #11622 ) ;
#5934=CIRCLE ( 'NONE', #1804, 3.000000000000000000 ) ;
#5949=CARTESIAN_POINT ( 'NONE',  ( -7.497885806132468467, -44.50611869254105102, 18.00659976627173720 ) ) ;
#5952=LINE ( 'NONE', #9323, #3576 ) ;
#5956=CIRCLE ( 'NONE', #10355, 10.00000000000000000 ) ;
#5957=CARTESIAN_POINT ( 'NONE',  ( -23.49969986081099904, -44.50737899243799944, -5.497689735156002122 ) ) ;
#5963=ORIENTED_EDGE ( 'NONE', *, *, #14486, .F. ) ;
#5972=DIRECTION ( 'NONE',  ( 0.000000000000000000, 0.000000000000000000, 1.000000000000000000 ) ) ;
#5974=ADVANCED_FACE ( 'NONE', ( #7953 ), #5369, .F. ) ;
#5978=CARTESIAN_POINT ( 'NONE',  ( 4.376462137075568748, -38.10176464241877881, -12.29701886598900806 ) ) ;
#5980=ORIENTED_EDGE ( 'NONE', *, *, #13810, .F. ) ;
#5986=ORIENTED_EDGE ( 'NONE', *, *, #1585, .F. ) ;
#5995=ORIENTED_EDGE ( 'NONE', *, *, #7360, .T. ) ;
#6001=AXIS2_PLACEMENT_3D ( 'NONE', #4013, #11271, #12497 ) ;
#6006=CARTESIAN_POINT ( 'NONE',  ( -23.49969986081099904, -44.50737899243799944, 19.50231026484399877 ) ) ;
#6015=CARTESIAN_POINT ( 'NONE',  ( -15.42469986081099442, -23.50737899243800300, 56.85231026484400019 ) ) ;
#6016=PLANE ( 'NONE',  #12665 ) ;
#6030=CARTESIAN_POINT ( 'NONE',  ( -33.49969986081094220, -41.82625798754038016, -13.39525803434798412 ) ) ;
#6041=AXIS2_PLACEMENT_3D ( 'NONE', #7058, #11736, #128 ) ;
#6043=EDGE_CURVE ( 'NONE', #8709, #2126, #4197, .T. ) ;
#6047=CARTESIAN_POINT ( 'NONE',  ( 2.500300139188999182, -42.00737899243800655, -13.39525803434800011 ) ) ;
#6056=CIRCLE ( 'NONE', #1432, 37.50000000000000000 ) ;
#6061=EDGE_CURVE ( 'NONE', #12214, #2702, #11139, .T. ) ;
#6063=CARTESIAN_POINT ( 'NONE',  ( -7.526618194427104669, -48.92257192762266271, -6.159325076304092761 ) ) ;
#6073=VECTOR ( 'NONE', #411, 1000.000000000000000 ) ;
#6074=CARTESIAN_POINT ( 'NONE',  ( -12.91616447596942230, -36.91800560015940391, -17.91172472810691119 ) ) ;
#6076=DIRECTION ( 'NONE',  ( 0.000000000000000000, 1.000000000000000000, 1.224646799147350002E-16 ) ) ;
#6080=AXIS2_PLACEMENT_3D ( 'NONE', #13752, #900, #1050 ) ;
#6082=DIRECTION ( 'NONE',  ( 0.000000000000000000, -1.000000000000000000, -1.224646799147350002E-16 ) ) ;
#6083=ORIENTED_EDGE ( 'NONE', *, *, #5377, .T. ) ;
#6100=CARTESIAN_POINT ( 'NONE',  ( -15.49969986081099194, -57.00737899243800655, 19.50231026484399521 ) ) ;
#6103=CARTESIAN_POINT ( 'NONE',  ( -7.510312366833470143, -44.09314884015893199, -4.806344695767887920 ) ) ;
#6110=EDGE_LOOP ( 'NONE', ( #2830, #10989, #7686, #12237 ) ) ;
#6133=CIRCLE ( 'NONE', #11531, 2.999999999999999112 ) ;
#6136=CARTESIAN_POINT ( 'NONE',  ( -7.513186133687160151, -48.97671528745701863, -5.011691156799132685 ) ) ;
#6158=CARTESIAN_POINT ( 'NONE',  ( -7.497885806132468467, -44.50611869254105102, 18.00659976627173720 ) ) ;
#6163=DIRECTION ( 'NONE',  ( 1.000000000000000000, 0.000000000000000000, 0.000000000000000000 ) ) ;
#6166=CARTESIAN_POINT ( 'NONE',  ( -7.497219220929387973, -44.39058125335130001, 18.15858026693495475 ) ) ;
#6178=AXIS2_PLACEMENT_3D ( 'NONE', #13070, #6082, #10841 ) ;
#6181=CARTESIAN_POINT ( 'NONE',  ( -12.19394264074465895, -51.79708643885629726, -17.85247874086887165 ) ) ;
#6207=DIRECTION ( 'NONE',  ( 0.000000000000000000, -1.000000000000000000, -1.224646799147350002E-16 ) ) ;
#6217=CARTESIAN_POINT ( 'NONE',  ( -7.638565634192135079, -48.52246210453047581, -4.016914597510680807 ) ) ;
#6220=CARTESIAN_POINT ( 'NONE',  ( -15.49969986081099371, -52.50737899243799944, -17.99768973515599768 ) ) ;
#6223=ORIENTED_EDGE ( 'NONE', *, *, #12788, .T. ) ;
#6224=CARTESIAN_POINT ( 'NONE',  ( -23.08909483861678069, -47.09084248276676732, 56.22686388828775961 ) ) ;
#6231=ORIENTED_EDGE ( 'NONE', *, *, #12022, .F. ) ;
#6239=CARTESIAN_POINT ( 'NONE',  ( -29.57393575939416408, -54.93314309385483796, 54.32987364559346588 ) ) ;
#6248=B_SPLINE_CURVE_WITH_KNOTS ( 'NONE', 3,
 ( #6983, #10525, #2572, #3718, #8147, #3795, #8223, #8454, #3489, #8374, #9605, #13063, #53, #12838, #11902, #3566, #6914, #6074, #10758, #281, #4721, #2273 ),
 .UNSPECIFIED., .F., .F.,
 ( 4, 2, 2, 2, 2, 2, 2, 2, 2, 2, 4 ),
 ( 0.000000000000000000, 0.001575913261410275554, 0.002363869892115413440, 0.003151826522820551108, 0.004727739784230826879, 0.006303653045641103084, 0.007091609676346248559, 0.007879566307051392299, 0.009455479568461672840, 0.01103139282987195165, 0.01260730609128223219 ),
 .UNSPECIFIED. ) ;
#6251=CARTESIAN_POINT ( 'NONE',  ( -14.45576569028314218, -52.45646407435158665, -17.98672605992057072 ) ) ;
#6255=ORIENTED_EDGE ( 'NONE', *, *, #14579, .F. ) ;
#6258=CARTESIAN_POINT ( 'NONE',  ( -36.51509609678214474, -37.41693849659213811, -11.55597063191085283 ) ) ;
#6259=ORIENTED_EDGE ( 'NONE', *, *, #4819, .T. ) ;
#6261=ADVANCED_BREP_SHAPE_REPRESENTATION ( '', ( #12764, #6789 ), #14627 ) ;
#6275=CARTESIAN_POINT ( 'NONE',  ( -7.504258367036227284, -44.23032460206619731, 45.54293165267414878 ) ) ;
#6276=DIRECTION ( 'NONE',  ( 0.000000000000000000, 0.000000000000000000, 1.000000000000000000 ) ) ;
#6282=ORIENTED_EDGE ( 'NONE', *, *, #3434, .T. ) ;
#6285=ORIENTED_EDGE ( 'NONE', *, *, #6831, .F. ) ;
#6299=CARTESIAN_POINT ( 'NONE',  ( -23.24400209454358901, -46.58079323946816430, 56.19408944517149962 ) ) ;
#6306=CARTESIAN_POINT ( 'NONE',  ( -8.489236575244433425, -20.67953079448830422, 56.34577682959393741 ) ) ;
#6315=ORIENTED_EDGE ( 'NONE', *, *, #8192, .F. ) ;
#6333=ORIENTED_EDGE ( 'NONE', *, *, #7932, .F. ) ;
#6334=CARTESIAN_POINT ( 'NONE',  ( 2.500300139188998738, -46.50737899243799944, 47.00231026484399877 ) ) ;
#6343=EDGE_CURVE ( 'NONE', #10539, #2418, #4648, .T. ) ;
#6346=EDGE_CURVE ( 'NONE', #1229, #6874, #6376, .T. ) ;
#6349=LINE ( 'NONE', #1620, #1747 ) ;
#6363=DIRECTION ( 'NONE',  ( 1.000000000000000000, 0.000000000000000000, 0.000000000000000000 ) ) ;
#6370=ORIENTED_EDGE ( 'NONE', *, *, #11309, .F. ) ;
#6376=B_SPLINE_CURVE_WITH_KNOTS ( 'NONE', 3,
 ( #2355, #11675, #5851, #10529, #2803, #10985, #10837, #1651, #12132, #1505, #9839, #8610, #13362, #9686, #14359, #14578, #7532, #7305, #13297, #437, #7455, #3798, #5027, #2578, #5248, #11987, #10909, #6306, #3874, #1431 ),
 .UNSPECIFIED., .F., .F.,
 ( 4, 2, 2, 2, 1, 1, 1, 1, 2, 2, 2, 2, 2, 1, 1, 2, 2, 4 ),
 ( 0.000000000000000000, 0.2500000000000077161, 0.3750000000000112688, 0.4375000000000130451, 0.4687500000000140443, 0.4843750000000142664, 0.4921875000000144329, 0.4960937500000142664, 0.4980468750000140443, 0.5000000000000137668, 0.6250000000000028866, 0.6874999999999971134, 0.7187499999999943379, 0.7343749999999925615, 0.7421874999999923395, 0.7460937499999922284, 0.7499999999999921174, 1.000000000000000000 ),
 .UNSPECIFIED. ) ;
#6380=PLANE ( 'NONE',  #4090 ) ;
#6388=ORIENTED_EDGE ( 'NONE', *, *, #13359, .F. ) ;
#6395=CARTESIAN_POINT ( 'NONE',  ( -7.500433020662215178, -49.00523987278725713, 19.39053537552759821 ) ) ;
#6403=CARTESIAN_POINT ( 'NONE',  ( -7.501944906337848273, -44.50613385756380325, -4.001965388595783324 ) ) ;
#6407=CARTESIAN_POINT ( 'NONE',  ( -35.39631831511088222, -38.07367433585212524, -12.28530471890510434 ) ) ;
#6409=ORIENTED_EDGE ( 'NONE', *, *, #15036, .F. ) ;
#6416=DIRECTION ( 'NONE',  ( -1.000000000000000000, 1.291538348938060198E-32, -1.054621095516909827E-16 ) ) ;
#6418=DIRECTION ( 'NONE',  ( 1.000000000000000000, -1.291538348938060198E-32, 1.054621095516909827E-16 ) ) ;
#6426=CARTESIAN_POINT ( 'NONE',  ( -7.497874475122997318, -44.50608669435617770, -6.993290823733421036 ) ) ;
#6430=DIRECTION ( 'NONE',  ( 0.000000000000000000, 1.850371707708594316E-16, -1.000000000000000000 ) ) ;
#6448=CARTESIAN_POINT ( 'NONE',  ( -20.38837171516173186, -50.86174603611942757, 56.68489931584038288 ) ) ;
#6450=CARTESIAN_POINT ( 'NONE',  ( -15.49969986081099904, -36.50737899243799944, 57.00231026484399877 ) ) ;
#6455=DIRECTION ( 'NONE',  ( 1.000000000000000000, 0.000000000000000000, 0.000000000000000000 ) ) ;
#6464=ORIENTED_EDGE ( 'NONE', *, *, #14642, .T. ) ;
#6472=ORIENTED_EDGE ( 'NONE', *, *, #7482, .T. ) ;
#6475=CARTESIAN_POINT ( 'NONE',  ( -7.742611511953769288, -46.45389122984595076, -2.997689585474093477 ) ) ;
#6477=CARTESIAN_POINT ( 'NONE',  ( -37.90618493125413124, -37.00737899243799234, -10.57698671581674077 ) ) ;
#6479=ORIENTED_EDGE ( 'NONE', *, *, #9342, .F. ) ;
#6488=DIRECTION ( 'NONE',  ( 0.000000000000000000, 0.000000000000000000, -1.000000000000000000 ) ) ;
#6489=CARTESIAN_POINT ( 'NONE',  ( -15.42469993581076970, -23.50709773904532085, 57.00223526491900117 ) ) ;
#6495=CARTESIAN_POINT ( 'NONE',  ( 4.000300139189000959, -19.50737899243798879, -17.99768973515599768 ) ) ;
#6497=ORIENTED_EDGE ( 'NONE', *, *, #13423, .F. ) ;
#6509=CARTESIAN_POINT ( 'NONE',  ( -7.753733168396170328, -46.50737899243799944, 47.00231026484399877 ) ) ;
#6510=AXIS2_PLACEMENT_3D ( 'NONE', #2072, #6418, #10091 ) ;
#6512=VERTEX_POINT ( 'NONE', #11137 ) ;
#6515=VERTEX_POINT ( 'NONE', #7608 ) ;
#6527=VECTOR ( 'NONE', #13646, 1000.000000000000000 ) ;
#6548=( BOUNDED_CURVE ( )  B_SPLINE_CURVE ( 3, ( #14807, #14885, #11366, #13814 ),
 .UNSPECIFIED., .F., .F. ) 
 B_SPLINE_CURVE_WITH_KNOTS ( ( 4, 4 ),
 ( 5.024656459356720006, 6.283185307179586232 ),
 .UNSPECIFIED. ) 
 CURVE ( )  GEOMETRIC_REPRESENTATION_ITEM ( )  RATIONAL_B_SPLINE_CURVE ( ( 1.000000000000000000, 0.8723071003127500500, 0.8723071003127500500, 1.000000000000000000 ) ) 
 REPRESENTATION_ITEM ( '' )  );
#6550=LINE ( 'NONE', #10072, #6932 ) ;
#6559=CARTESIAN_POINT ( 'NONE',  ( -15.49969986081099016, -52.50737899243799944, 27.50231026484399521 ) ) ;
#6560=CARTESIAN_POINT ( 'NONE',  ( -9.141872392333175057, -49.39150629834951900, 56.46061503045971364 ) ) ;
#6563=CARTESIAN_POINT ( 'NONE',  ( -8.492287438043703673, -48.36911050528196654, 42.82612708017594372 ) ) ;
#6565=CARTESIAN_POINT ( 'NONE',  ( -15.49969986081099371, -57.00737899243799944, -17.99768973515599768 ) ) ;
#6567=CIRCLE ( 'NONE', #231, 37.50000000000000000 ) ;
#6568=CARTESIAN_POINT ( 'NONE',  ( -7.512147529361665299, -44.06076409293740426, 45.03331134192608687 ) ) ;
#6573=ORIENTED_EDGE ( 'NONE', *, *, #4513, .F. ) ;
#6576=ORIENTED_EDGE ( 'NONE', *, *, #8508, .T. ) ;
#6577=FACE_OUTER_BOUND ( 'NONE', #13173, .T. ) ;
#6579=VECTOR ( 'NONE', #11581, 1000.000000000000000 ) ;
#6580=CARTESIAN_POINT ( 'NONE',  ( -7.821533452792987617, -47.59505538333905150, -7.749013365421348887 ) ) ;
#6583=CARTESIAN_POINT ( 'NONE',  ( -5.499699860811000818, -46.50737899243799944, 16.50231026484399877 ) ) ;
#6612=CARTESIAN_POINT ( 'NONE',  ( -15.49969986081099194, -27.00737899243800300, 19.50231026484399877 ) ) ;
#6623=DIRECTION ( 'NONE',  ( 0.000000000000000000, 0.000000000000000000, 1.000000000000000000 ) ) ;
#6631=VERTEX_POINT ( 'NONE', #7033 ) ;
#6636=FACE_OUTER_BOUND ( 'NONE', #5171, .T. ) ;
#6644=ORIENTED_EDGE ( 'NONE', *, *, #8424, .F. ) ;
#6647=ORIENTED_EDGE ( 'NONE', *, *, #3956, .T. ) ;
#6650=ORIENTED_EDGE ( 'NONE', *, *, #12432, .F. ) ;
#6654=ORIENTED_EDGE ( 'NONE', *, *, #960, .F. ) ;
#6656=LINE ( 'NONE', #11339, #2575 ) ;
#6657=CARTESIAN_POINT ( 'NONE',  ( -15.49969986081099016, -36.50737899243799944, 27.50231026484399521 ) ) ;
#6663=CARTESIAN_POINT ( 'NONE',  ( -32.87150473820536689, -24.05954647699559601, -13.82452877272130642 ) ) ;
#6666=ORIENTED_EDGE ( 'NONE', *, *, #5048, .F. ) ;
#6667=CARTESIAN_POINT ( 'NONE',  ( 2.500300139188996518, -46.50737899243799944, 44.50231026484399877 ) ) ;
#6670=CARTESIAN_POINT ( 'NONE',  ( 2.500300139188999182, -42.00737899243800655, 52.39987856403599409 ) ) ;
#6678=CARTESIAN_POINT ( 'NONE',  ( -7.742536611909244471, -46.45380687591467250, 22.00231042132131165 ) ) ;
#6679=PLANE ( 'NONE',  #9858 ) ;
#6701=ORIENTED_EDGE ( 'NONE', *, *, #5854, .T. ) ;
#6703=CARTESIAN_POINT ( 'NONE',  ( -20.18599136182625742, -52.50737899243802786, -13.49768973515603676 ) ) ;
#6709=CARTESIAN_POINT ( 'NONE',  ( -10.21738681012386429, -50.52121012465195093, 56.62897346558520439 ) ) ;
#6717=VERTEX_POINT ( 'NONE', #11018 ) ;
#6720=DIRECTION ( 'NONE',  ( 0.000000000000000000, 0.000000000000000000, 1.000000000000000000 ) ) ;
#6722=VERTEX_POINT ( 'NONE', #546 ) ;
#6730=EDGE_CURVE ( 'NONE', #12928, #1528, #7019, .T. ) ;
#6733=CARTESIAN_POINT ( 'NONE',  ( -7.797100586692802260, -47.75470106918066193, -7.664321372934788990 ) ) ;
#6735=VERTEX_POINT ( 'NONE', #9729 ) ;
#6741=CARTESIAN_POINT ( 'NONE',  ( 2.656674150012286351, -40.75537920817077975, 52.31386353015493285 ) ) ;
#6750=CARTESIAN_POINT ( 'NONE',  ( -7.586208288801848276, -45.66796403488923772, 21.86702897299116088 ) ) ;
#6753=VERTEX_POINT ( 'NONE', #14545 ) ;
#6760=CARTESIAN_POINT ( 'NONE',  ( -23.43465585259791695, -43.45604609243036265, 56.15319261074063206 ) ) ;
#6768=CARTESIAN_POINT ( 'NONE',  ( -7.499706911750000593, -49.00740941973811005, 19.72872175748142709 ) ) ;
#6784=CARTESIAN_POINT ( 'NONE',  ( -11.02342383152547178, -36.50737899243796392, 2.502310264844030296 ) ) ;
#6785=CARTESIAN_POINT ( 'NONE',  ( -13.42547148602778684, -52.23827942061129193, 56.94575044587081436 ) ) ;
#6789=AXIS2_PLACEMENT_3D ( 'NONE', #4381, #12419, #6809 ) ;
#6792=DIRECTION ( 'NONE',  ( 0.000000000000000000, 0.000000000000000000, 1.000000000000000000 ) ) ;
#6797=ORIENTED_EDGE ( 'NONE', *, *, #7474, .T. ) ;
#6799=VERTEX_POINT ( 'NONE', #1444 ) ;
#6801=PRODUCT_DEFINITION_FORMATION_WITH_SPECIFIED_SOURCE ( 'ANY', '', #11171, .NOT_KNOWN. ) ;
#6802=ADVANCED_FACE ( 'NONE', ( #3811 ), #6016, .T. ) ;
#6809=DIRECTION ( 'NONE',  ( 1.000000000000000000, 0.000000000000000000, 0.000000000000000000 ) ) ;
#6810=AXIS2_PLACEMENT_3D ( 'NONE', #12646, #12722, #1084 ) ;
#6813=ORIENTED_EDGE ( 'NONE', *, *, #393, .F. ) ;
#6815=EDGE_LOOP ( 'NONE', ( #6255, #2674, #5885, #14335, #8165, #5532, #12546, #6282 ) ) ;
#6818=( BOUNDED_CURVE ( )  B_SPLINE_CURVE ( 3, ( #11656, #1036, #12509, #1104 ),
 .UNSPECIFIED., .F., .F. ) 
 B_SPLINE_CURVE_WITH_KNOTS ( ( 4, 4 ),
 ( 4.712388980384689674, 6.283185307179586232 ),
 .UNSPECIFIED. ) 
 CURVE ( )  GEOMETRIC_REPRESENTATION_ITEM ( )  RATIONAL_B_SPLINE_CURVE ( ( 1.000000000000000000, 0.8047378541243649375, 0.8047378541243649375, 1.000000000000000000 ) ) 
 REPRESENTATION_ITEM ( '' )  );
#6827=CARTESIAN_POINT ( 'NONE',  ( -7.499699860810998153, -43.98402112729824864, 56.13904046828872652 ) ) ;
#6828=B_SPLINE_CURVE_WITH_KNOTS ( 'NONE', 3,
 ( #7079, #13078, #4809, #1210, #3736, #7318 ),
 .UNSPECIFIED., .F., .F.,
 ( 4, 2, 4 ),
 ( 0.000000000000000000, 0.1441277441444622220, 0.2882554882889244441 ),
 .UNSPECIFIED. ) ;
#6831=EDGE_CURVE ( 'NONE', #3128, #11105, #11360, .T. ) ;
#6834=FACE_OUTER_BOUND ( 'NONE', #4128, .T. ) ;
#6839=CARTESIAN_POINT ( 'NONE',  ( -34.99969986081099904, -19.50737899243800300, 51.22375411596780026 ) ) ;
#6842=ORIENTED_EDGE ( 'NONE', *, *, #4592, .F. ) ;
#6847=EDGE_CURVE ( 'NONE', #14890, #8709, #11847, .T. ) ;
#6863=DIRECTION ( 'NONE',  ( 1.000000000000000000, -1.291538348938060198E-32, 1.054621095516909827E-16 ) ) ;
#6865=ADVANCED_FACE ( 'NONE', ( #14221 ), #13082, .T. ) ;
#6874=VERTEX_POINT ( 'NONE', #7320 ) ;
#6886=CARTESIAN_POINT ( 'NONE',  ( -22.67629672040707334, -48.05217323185801348, -17.30478718853205322 ) ) ;
#6891=CARTESIAN_POINT ( 'NONE',  ( -23.49969986081099904, -19.50737899243800300, 48.00231026484399877 ) ) ;
#6895=ORIENTED_EDGE ( 'NONE', *, *, #9247, .F. ) ;
#6896=EDGE_CURVE ( 'NONE', #5522, #12480, #6656, .T. ) ;
#6897=CARTESIAN_POINT ( 'NONE',  ( -21.33331128615267858, -21.63851970382446055, 56.54902971347384266 ) ) ;
#6899=DIRECTION ( 'NONE',  ( 0.000000000000000000, 0.000000000000000000, -1.000000000000000000 ) ) ;
#6909=ORIENTED_EDGE ( 'NONE', *, *, #8063, .F. ) ;
#6913=CARTESIAN_POINT ( 'NONE',  ( -15.49969986081099904, -57.00737899243800655, -5.497689735156002122 ) ) ;
#6914=CARTESIAN_POINT ( 'NONE',  ( -11.95055483344002312, -37.31872034517681413, -17.83250243206357410 ) ) ;
#6919=( GEOMETRIC_REPRESENTATION_CONTEXT ( 3 ) GLOBAL_UNCERTAINTY_ASSIGNED_CONTEXT ( ( #11988 ) ) GLOBAL_UNIT_ASSIGNED_CONTEXT ( ( #14278, #1265, #208 ) ) REPRESENTATION_CONTEXT ( 'NONE', 'WORKASPACE' ) );
#6922=CARTESIAN_POINT ( 'NONE',  ( -7.501950027729723303, -44.50597529135383468, 20.99749114769749880 ) ) ;
#6930=CARTESIAN_POINT ( 'NONE',  ( -7.704540658288731692, -46.31685722003375361, 47.00231026484399166 ) ) ;
#6932=VECTOR ( 'NONE', #12535, 1000.000000000000000 ) ;
#6934=DIRECTION ( 'NONE',  ( -1.000000000000000000, 1.291538348938060198E-32, -1.054621095516909827E-16 ) ) ;
#6957=CARTESIAN_POINT ( 'NONE',  ( 7.203956337210061456, -37.00737899243799944, -10.34622021768276667 ) ) ;
#6958=ORIENTED_EDGE ( 'NONE', *, *, #3691, .F. ) ;
#6963=CARTESIAN_POINT ( 'NONE',  ( 4.127468730679389353, -38.31628777932305496, 51.45578572424146557 ) ) ;
#6968=DIRECTION ( 'NONE',  ( 1.000000000000000000, 0.000000000000000000, 0.000000000000000000 ) ) ;
#6970=B_SPLINE_CURVE_WITH_KNOTS ( 'NONE', 3,
 ( #9547, #3091, #7603, #1801 ),
 .UNSPECIFIED., .F., .F.,
 ( 4, 4 ),
 ( 0.8772494290945609396, 1.000000000000000000 ),
 .UNSPECIFIED. ) ;
#6971=CARTESIAN_POINT ( 'NONE',  ( -7.507587349371155128, -44.88838417754359966, 21.40739837630950504 ) ) ;
#6982=ORIENTED_EDGE ( 'NONE', *, *, #13441, .T. ) ;
#6983=CARTESIAN_POINT ( 'NONE',  ( -7.499699860810999041, -44.50737899243799944, -17.13441993860073964 ) ) ;
#6992=CARTESIAN_POINT ( 'NONE',  ( -38.49969986081099904, -37.00737899243799944, 52.39987856403599409 ) ) ;
#7004=FACE_BOUND ( 'NONE', #11820, .T. ) ;
#7009=CARTESIAN_POINT ( 'NONE',  ( -11.02342383152546645, -36.50737899243797102, 11.50231026484397034 ) ) ;
#7010=B_SPLINE_CURVE_WITH_KNOTS ( 'NONE', 3,
 ( #4386, #9039, #2091, #14074, #3517, #6580, #944, #12344, #9406, #6733, #11265, #4668, #9324, #12861, #2376, #7013, #1862, #5873, #2786, #10592, #14268, #7288, #7441, #6063, #8592, #4864, #1412, #9517, #125, #3785, #424, #2562, #7210, #6136, #1255, #5913, #8365, #10745, #10823, #6217, #11890, #14111, #4785, #4935, #1490, #272, #8286, #14344, #9442 ),
 .UNSPECIFIED., .F., .F.,
 ( 4, 2, 2, 1, 1, 2, 2, 2, 2, 1, 1, 2, 2, 2, 2, 2, 1, 2, 2, 2, 2, 2, 1, 1, 2, 2, 2, 4 ),
 ( 0.000000000000000000, 0.06250000000000491274, 0.09375000000000881240, 0.1093750000000107969, 0.1171875000000118239, 0.1210937500000123374, 0.1250000000000128508, 0.1875000000000081324, 0.2187500000000046074, 0.2343750000000028866, 0.2421875000000020539, 0.2460937500000008049, 0.2499999999999995559, 0.3750000000000037192, 0.4375000000000054401, 0.4687500000000063838, 0.4843750000000064948, 0.4921875000000063283, 0.5000000000000061062, 0.6250000000000033307, 0.6875000000000025535, 0.7187500000000021094, 0.7343750000000025535, 0.7421875000000033307, 0.7460937500000037748, 0.7500000000000042188, 0.8750000000000021094, 1.000000000000000000 ),
 .UNSPECIFIED. ) ;
#7013=CARTESIAN_POINT ( 'NONE',  ( -7.690624001723991299, -48.30857337213005565, -7.231759084041137875 ) ) ;
#7016=CARTESIAN_POINT ( 'NONE',  ( -35.59468245696151456, -37.93213861349480709, 51.16428679575325589 ) ) ;
#7019=CIRCLE ( 'NONE', #12418, 10.00000000000000000 ) ;
#7022=ORIENTED_EDGE ( 'NONE', *, *, #7342, .F. ) ;
#7029=DIRECTION ( 'NONE',  ( 1.054621095516909827E-16, 1.224646799147350002E-16, -1.000000000000000000 ) ) ;
#7033=CARTESIAN_POINT ( 'NONE',  ( -7.499699860810999041, -44.50737899243799944, 43.00231026484400587 ) ) ;
#7040=CARTESIAN_POINT ( 'NONE',  ( 2.995488256399623239, -39.83604612058397976, -13.11945893988026413 ) ) ;
#7043=ORIENTED_EDGE ( 'NONE', *, *, #6831, .T. ) ;
#7044=B_SPLINE_CURVE_WITH_KNOTS ( 'NONE', 3,
 ( #3962, #521, #14591, #14372 ),
 .UNSPECIFIED., .F., .F.,
 ( 4, 4 ),
 ( 0.000000000000000000, 0.1210918566152707487 ),
 .UNSPECIFIED. ) ;
#7058=CARTESIAN_POINT ( 'NONE',  ( -15.49969986081099904, -27.00737899243800300, -5.497689735156002122 ) ) ;
#7060=ORIENTED_EDGE ( 'NONE', *, *, #1585, .T. ) ;
#7062=CARTESIAN_POINT ( 'NONE',  ( -23.23036473679183445, -42.43240574409319521, 56.19689949488600433 ) ) ;
#7077=CARTESIAN_POINT ( 'NONE',  ( -27.49969986081100259, -57.00737899243800655, 19.50231026484398811 ) ) ;
#7078=ORIENTED_EDGE ( 'NONE', *, *, #14406, .F. ) ;
#7079=CARTESIAN_POINT ( 'NONE',  ( -7.512805849530849400, -44.04964101872670312, -5.955427708867301106 ) ) ;
#7086=DIRECTION ( 'NONE',  ( 0.000000000000000000, 0.000000000000000000, -1.000000000000000000 ) ) ;
#7092=LINE ( 'NONE', #11775, #11416 ) ;
#7103=VERTEX_POINT ( 'NONE', #2688 ) ;
#7116=CARTESIAN_POINT ( 'NONE',  ( 5.799466111164440996, -37.30547240248169771, -11.36184443632733654 ) ) ;
#7121=VECTOR ( 'NONE', #9679, 1000.000000000000000 ) ;
#7128=VECTOR ( 'NONE', #13820, 1000.000000000000000 ) ;
#7131=( BOUNDED_CURVE ( )  B_SPLINE_CURVE ( 3, ( #10687, #9539, #14208, #9391 ),
 .UNSPECIFIED., .F., .T. ) 
 B_SPLINE_CURVE_WITH_KNOTS ( ( 4, 4 ),
 ( 1.023945376098953641, 1.222940073837788466 ),
 .UNSPECIFIED. ) 
 CURVE ( )  GEOMETRIC_REPRESENTATION_ITEM ( )  RATIONAL_B_SPLINE_CURVE ( ( 1.000000000000000000, 0.9967028139718016044, 0.9967028139718016044, 1.000000000000000000 ) ) 
 REPRESENTATION_ITEM ( '' )  );
#7132=VECTOR ( 'NONE', #11374, 1000.000000000000000 ) ;
#7142=CARTESIAN_POINT ( 'NONE',  ( -21.86069005650799468, -39.62793443228212453, 56.46004693087562032 ) ) ;
#7144=SURFACE_STYLE_USAGE ( .BOTH. , #2490 ) ;
#7196=CARTESIAN_POINT ( 'NONE',  ( 2.540007305964766093, -41.28381732925497971, -13.37362536790431022 ) ) ;
#7200=AXIS2_PLACEMENT_3D ( 'NONE', #9549, #12936, #2444 ) ;
#7202=VERTEX_POINT ( 'NONE', #1465 ) ;
#7210=CARTESIAN_POINT ( 'NONE',  ( -7.499706911750001481, -49.00740941973812426, -5.271278242526713953 ) ) ;
#7218=CARTESIAN_POINT ( 'NONE',  ( -23.07797347600723015, -41.93085761288553215, 56.22867446278029036 ) ) ;
#7221=( BOUNDED_CURVE ( )  B_SPLINE_CURVE ( 3, ( #9049, #8973, #1099, #11503 ),
 .UNSPECIFIED., .F., .T. ) 
 B_SPLINE_CURVE_WITH_KNOTS ( ( 4, 4 ),
 ( 6.505213034913054214E-16, 1.513547814233603184 ),
 .UNSPECIFIED. ) 
 CURVE ( )  GEOMETRIC_REPRESENTATION_ITEM ( )  RATIONAL_B_SPLINE_CURVE ( ( 1.000000000000000000, 0.8180365063541295001, 0.8180365063541295001, 1.000000000000000000 ) ) 
 REPRESENTATION_ITEM ( '' )  );
#7223=LINE ( 'NONE', #1575, #13437 ) ;
#7225=CARTESIAN_POINT ( 'NONE',  ( -7.541204214081353108, -45.30969539143143976, 17.30566581272957905 ) ) ;
#7229=VERTEX_POINT ( 'NONE', #8867 ) ;
#7230=EDGE_CURVE ( 'NONE', #777, #5522, #11392, .T. ) ;
#7231=CARTESIAN_POINT ( 'NONE',  ( -7.512805849530849400, -44.04964101872670312, 19.04457229113268113 ) ) ;
#7239=AXIS2_PLACEMENT_3D ( 'NONE', #7571, #6416, #13181 ) ;
#7241=VECTOR ( 'NONE', #8544, 1000.000000000000000 ) ;
#7243=ORIENTED_EDGE ( 'NONE', *, *, #214, .T. ) ;
#7244=DIRECTION ( 'NONE',  ( 0.000000000000000000, 0.000000000000000000, 1.000000000000000000 ) ) ;
#7245=CARTESIAN_POINT ( 'NONE',  ( -34.11203994331643230, -39.60748137432106830, 52.05738518461070896 ) ) ;
#7262=AXIS2_PLACEMENT_3D ( 'NONE', #14492, #4012, #1566 ) ;
#7267=ADVANCED_FACE ( 'NONE', ( #6636 ), #14767, .T. ) ;
#7268=CARTESIAN_POINT ( 'NONE',  ( 4.269688099973369511, -38.19079675818824882, -12.36340031411550733 ) ) ;
#7273=ORIENTED_EDGE ( 'NONE', *, *, #9140, .T. ) ;
#7276=EDGE_CURVE ( 'NONE', #10198, #11004, #7677, .T. ) ;
#7288=CARTESIAN_POINT ( 'NONE',  ( -7.607412389351755344, -48.63717025145610506, -6.846874655572149138 ) ) ;
#7291=VECTOR ( 'NONE', #9443, 1000.000000000000000 ) ;
#7297=ORIENTED_EDGE ( 'NONE', *, *, #12542, .F. ) ;
#7304=DIRECTION ( 'NONE',  ( 0.000000000000000000, -1.850371707708594563E-16, 1.000000000000000000 ) ) ;
#7305=CARTESIAN_POINT ( 'NONE',  ( -9.919921220328577149, -21.80813450786784102, 56.58478691063636035 ) ) ;
#7318=CARTESIAN_POINT ( 'NONE',  ( -7.497874475122997318, -44.50608669435617770, -6.993290823733421036 ) ) ;
#7320=CARTESIAN_POINT ( 'NONE',  ( -7.499699860810999041, -19.50737899243799589, 56.13904046828879757 ) ) ;
#7324=CARTESIAN_POINT ( 'NONE',  ( -7.821533452793039132, -47.59505538333821306, 17.25098663457825410 ) ) ;
#7328=DIRECTION ( 'NONE',  ( 1.000000000000000000, 0.000000000000000000, 0.000000000000000000 ) ) ;
#7333=CARTESIAN_POINT ( 'NONE',  ( -7.753733168396166775, -46.50737899243799944, 42.00231026484399166 ) ) ;
#7340=ORIENTED_EDGE ( 'NONE', *, *, #9594, .T. ) ;
#7342=EDGE_CURVE ( 'NONE', #6753, #1019, #10452, .T. ) ;
#7353=CARTESIAN_POINT ( 'NONE',  ( -15.49969986081099904, -57.00737899243800655, 19.50231026484399877 ) ) ;
#7356=VECTOR ( 'NONE', #3077, 1000.000000000000000 ) ;
#7357=DIRECTION ( 'NONE',  ( 0.000000000000000000, -1.000000000000000000, -1.224646799147350002E-16 ) ) ;
#7360=EDGE_CURVE ( 'NONE', #10290, #11428, #3589, .T. ) ;
#7367=CARTESIAN_POINT ( 'NONE',  ( -20.18599136182624676, -52.50737899243804208, 11.50231026484396502 ) ) ;
#7372=CARTESIAN_POINT ( 'NONE',  ( -18.08681813700378171, -52.08207165106512093, 56.91381011686954849 ) ) ;
#7373=VERTEX_POINT ( 'NONE', #5949 ) ;
#7380=CYLINDRICAL_SURFACE ( 'NONE', #12205, 37.49999999999999289 ) ;
#7396=ORIENTED_EDGE ( 'NONE', *, *, #38, .T. ) ;
#7402=CARTESIAN_POINT ( 'NONE',  ( -7.501378586840248275, -49.00244658604240300, 19.34197447739098763 ) ) ;
#7408=CARTESIAN_POINT ( 'NONE',  ( -15.57469986081099478, -23.50709773848280904, 56.85231026484400019 ) ) ;
#7409=CARTESIAN_POINT ( 'NONE',  ( -7.505475668120653587, -44.32813276070414332, -4.257828788660135366 ) ) ;
#7411=CARTESIAN_POINT ( 'NONE',  ( -33.59815531783383591, -41.01804242337339446, -13.34120349808900130 ) ) ;
#7421=CARTESIAN_POINT ( 'NONE',  ( -7.795104587452824418, -46.66314860471634773, -2.997690171028501549 ) ) ;
#7432=CARTESIAN_POINT ( 'NONE',  ( -15.49969986081099727, -19.50737899243800300, 19.50231026484402008 ) ) ;
#7441=CARTESIAN_POINT ( 'NONE',  ( -7.567013331128950249, -48.78395362562350357, -6.570480905340088995 ) ) ;
#7445=ORIENTED_EDGE ( 'NONE', *, *, #10569, .F. ) ;
#7455=CARTESIAN_POINT ( 'NONE',  ( -9.418794693332646517, -21.44679481879670391, 56.50578474138158924 ) ) ;
#7459=ORIENTED_EDGE ( 'NONE', *, *, #4879, .F. ) ;
#7472=ADVANCED_FACE ( 'NONE', ( #15099, #13657 ), #4627, .F. ) ;
#7474=EDGE_CURVE ( 'NONE', #11428, #4941, #3671, .T. ) ;
#7475=CARTESIAN_POINT ( 'NONE',  ( -7.681929635180945404, -48.34577715838003087, 17.80744637252912455 ) ) ;
#7477=DIRECTION ( 'NONE',  ( 0.000000000000000000, 0.000000000000000000, 1.000000000000000000 ) ) ;
#7480=CARTESIAN_POINT ( 'NONE',  ( -33.49969986081093509, -41.64411882290328748, 52.39987856403602962 ) ) ;
#7482=EDGE_CURVE ( 'NONE', #13156, #3424, #10431, .T. ) ;
#7489=FACE_OUTER_BOUND ( 'NONE', #10809, .T. ) ;
#7493=CARTESIAN_POINT ( 'NONE',  ( -7.886584594865180264, -46.96511696614940234, -3.039951761444701361 ) ) ;
#7494=AXIS2_PLACEMENT_3D ( 'NONE', #3426, #4576, #10386 ) ;
#7499=AXIS2_PLACEMENT_3D ( 'NONE', #5172, #5326, #13366 ) ;
#7500=FACE_BOUND ( 'NONE', #13559, .T. ) ;
#7508=ORIENTED_EDGE ( 'NONE', *, *, #2141, .F. ) ;
#7531=ADVANCED_FACE ( 'NONE', ( #4780 ), #14338, .T. ) ;
#7532=CARTESIAN_POINT ( 'NONE',  ( -10.40142408276975594, -22.11861997768099641, 56.65522384219905661 ) ) ;
#7533=CARTESIAN_POINT ( 'NONE',  ( -15.42469986081099442, -26.50737899243800300, 56.85231026484400019 ) ) ;
#7547=VECTOR ( 'NONE', #7357, 1000.000000000000000 ) ;
#7567=VECTOR ( 'NONE', #12648, 1000.000000000000000 ) ;
#7571=CARTESIAN_POINT ( 'NONE',  ( 2.500300139188999182, -46.50737899243799944, 44.50231026484399877 ) ) ;
#7572=EDGE_CURVE ( 'NONE', #7870, #14077, #5, .T. ) ;
#7573=DIRECTION ( 'NONE',  ( 1.000000000000000000, 0.000000000000000000, 0.000000000000000000 ) ) ;
#7575=CARTESIAN_POINT ( 'NONE',  ( -7.515340199219564532, -44.00737819808650642, 44.63626335271796819 ) ) ;
#7579=ORIENTED_EDGE ( 'NONE', *, *, #13545, .F. ) ;
#7586=CARTESIAN_POINT ( 'NONE',  ( -15.49969986081099194, -27.00737899243800300, 19.50231026484399877 ) ) ;
#7588=CARTESIAN_POINT ( 'NONE',  ( -15.49969986081099727, -27.00737899243800300, 2.502310264843997878 ) ) ;
#7595=ORIENTED_EDGE ( 'NONE', *, *, #12266, .F. ) ;
#7596=DIRECTION ( 'NONE',  ( 0.000000000000000000, -1.000000000000000000, 0.000000000000000000 ) ) ;
#7603=CARTESIAN_POINT ( 'NONE',  ( -7.838474667259318629, -46.81609114312938402, -7.983182814980946063 ) ) ;
#7608=CARTESIAN_POINT ( 'NONE',  ( -34.99969986081099904, -20.37340439622244048, -12.52892449124999885 ) ) ;
#7611=ORIENTED_EDGE ( 'NONE', *, *, #2059, .F. ) ;
#7617=EDGE_LOOP ( 'NONE', ( #4540, #518 ) ) ;
#7618=CARTESIAN_POINT ( 'NONE',  ( -2.716578225681299141, -32.00737899243799944, -15.75165123257469801 ) ) ;
#7622=CARTESIAN_POINT ( 'NONE',  ( -7.662963790453772184, -48.42200951437349943, 17.89473638362698082 ) ) ;
#7624=CARTESIAN_POINT ( 'NONE',  ( -8.992083836519068285, -50.38952316532491693, -11.37983390804291517 ) ) ;
#7628=CARTESIAN_POINT ( 'NONE',  ( -7.694370900912546496, -46.24434200338747303, -3.010997809292743632 ) ) ;
#7632=ORIENTED_EDGE ( 'NONE', *, *, #1787, .F. ) ;
#7635=ORIENTED_EDGE ( 'NONE', *, *, #14783, .T. ) ;
#7636=VECTOR ( 'NONE', #14682, 1000.000000000000000 ) ;
#7639=CARTESIAN_POINT ( 'NONE',  ( -23.49969986081099904, -44.50737899243799944, -109.5506571639849938 ) ) ;
#7646=LINE ( 'NONE', #338, #2480 ) ;
#7652=ORIENTED_EDGE ( 'NONE', *, *, #13272, .F. ) ;
#7654=DIRECTION ( 'NONE',  ( -1.000000000000000000, -3.700743415417188632E-16, 0.000000000000000000 ) ) ;
#7669=ORIENTED_EDGE ( 'NONE', *, *, #515, .T. ) ;
#7670=ORIENTED_EDGE ( 'NONE', *, *, #5334, .F. ) ;
#7677=B_SPLINE_CURVE_WITH_KNOTS ( 'NONE', 3,
 ( #9167, #13696, #3211, #920, #12627, #7858, #12554, #1838, #5648, #6563, #5571, #14915, #9092, #14688, #13772, #3292, #7940, #10320, #4516, #11170, #4209, #3055, #7709, #1918, #11248, #5425, #9319, #5867, #11765, #1137, #10396, #229 ),
 .UNSPECIFIED., .F., .F.,
 ( 4, 2, 2, 2, 2, 2, 2, 2, 2, 2, 2, 2, 2, 2, 2, 4 ),
 ( 0.007859347252422295774, 0.008369889772020241286, 0.008880432291618185064, 0.009390974811216130577, 0.009901517330814076090, 0.01041205985041202160, 0.01092260237000996538, 0.01143314488960791089, 0.01194368740920585641, 0.01296477244840174570, 0.01347531496799970509, 0.01398585748759766448, 0.01449640000719562213, 0.01500694252679357979, 0.01551748504639154091, 0.01602802756598949857 ),
 .UNSPECIFIED. ) ;
#7686=ORIENTED_EDGE ( 'NONE', *, *, #2556, .F. ) ;
#7689=CARTESIAN_POINT ( 'NONE',  ( -15.49969986081100082, -19.50737899243800300, 19.50231026484399877 ) ) ;
#7703=CARTESIAN_POINT ( 'NONE',  ( -34.68185672695825872, -38.77348753601568632, -12.72054782938013062 ) ) ;
#7707=CARTESIAN_POINT ( 'NONE',  ( -7.704840168542555823, -46.32660887508429681, 56.18327162512064632 ) ) ;
#7709=CARTESIAN_POINT ( 'NONE',  ( -8.493401964816579053, -48.37115091595966732, 46.17630167696805898 ) ) ;
#7716=ADVANCED_FACE ( 'NONE', ( #5373 ), #8890, .T. ) ;
#7725=CARTESIAN_POINT ( 'NONE',  ( -28.28282149594069850, -32.00737899243799944, 54.75627176226269199 ) ) ;
#7728=LINE ( 'NONE', #12571, #240 ) ;
#7747=CARTESIAN_POINT ( 'NONE',  ( -12.91865582312666838, -36.91712645767735523, 56.91652338071235562 ) ) ;
#7751=EDGE_CURVE ( 'NONE', #9903, #14455, #941, .T. ) ;
#7757=CARTESIAN_POINT ( 'NONE',  ( 4.000300139189000959, -19.50737899243798879, -12.52892449124999885 ) ) ;
#7763=EDGE_LOOP ( 'NONE', ( #12886, #9759, #8504, #6409 ) ) ;
#7767=ORIENTED_EDGE ( 'NONE', *, *, #15036, .T. ) ;
#7768=LINE ( 'NONE', #14967, #7132 ) ;
#7770=PRODUCT_CONTEXT ( 'NONE', #10759, 'mechanical' ) ;
#7778=CARTESIAN_POINT ( 'NONE',  ( -23.49969986081099904, -44.50737899243799944, -5.497689735156002122 ) ) ;
#7779=ORIENTED_EDGE ( 'NONE', *, *, #12567, .F. ) ;
#7784=CARTESIAN_POINT ( 'NONE',  ( -12.92191964973194906, -52.08526088413143640, 56.91445648935585666 ) ) ;
#7800=ORIENTED_EDGE ( 'NONE', *, *, #7230, .F. ) ;
#7805=CYLINDRICAL_SURFACE ( 'NONE', #13477, 2.499999999999998668 ) ;
#7806=CARTESIAN_POINT ( 'NONE',  ( -28.28282149594069850, -32.00737899243799944, -15.75165123257469801 ) ) ;
#7811=VERTEX_POINT ( 'NONE', #6657 ) ;
#7813=CARTESIAN_POINT ( 'NONE',  ( -15.49969986081099016, -27.00737899243800300, 27.50231026484399877 ) ) ;
#7815=CARTESIAN_POINT ( 'NONE',  ( -7.552314780320042331, -43.45227698143176553, 56.15064027656714529 ) ) ;
#7817=ADVANCED_FACE ( 'NONE', ( #4610 ), #12573, .F. ) ;
#7828=ORIENTED_EDGE ( 'NONE', *, *, #10567, .F. ) ;
#7839=CARTESIAN_POINT ( 'NONE',  ( -7.869402401355066523, -47.25089185752115384, 21.90682449334191162 ) ) ;
#7842=CIRCLE ( 'NONE', #3955, 37.50000000000000000 ) ;
#7845=CARTESIAN_POINT ( 'NONE',  ( -7.506834498223213359, -44.86600688595157749, -3.611780095971914850 ) ) ;
#7852=CARTESIAN_POINT ( 'NONE',  ( 4.000300139189000959, -20.37340439622241917, -12.52892449124999885 ) ) ;
#7853=CARTESIAN_POINT ( 'NONE',  ( -14.96933016362806690, -52.50737899243799234, 57.00231026484399166 ) ) ;
#7858=CARTESIAN_POINT ( 'NONE',  ( -8.123284869591744339, -47.60801320870127995, 42.25191011081004433 ) ) ;
#7870=VERTEX_POINT ( 'NONE', #1156 ) ;
#7871=LINE ( 'NONE', #12563, #9698 ) ;
#7872=DIRECTION ( 'NONE',  ( 0.000000000000000000, -9.251858538542971581E-17, 1.000000000000000000 ) ) ;
#7886=ADVANCED_FACE ( 'NONE', ( #5889 ), #11637, .F. ) ;
#7887=CARTESIAN_POINT ( 'NONE',  ( -20.97295351809511388, -50.34796644937742371, -17.59659479099292412 ) ) ;
#7891=DIRECTION ( 'NONE',  ( 1.000000000000000000, -1.291538348938060198E-32, 1.054621095516909827E-16 ) ) ;
#7896=CARTESIAN_POINT ( 'NONE',  ( -11.26730675207693899, -37.71366398918802787, 56.76333939437698461 ) ) ;
#7911=VERTEX_POINT ( 'NONE', #8422 ) ;
#7912=ORIENTED_EDGE ( 'NONE', *, *, #7751, .F. ) ;
#7915=CARTESIAN_POINT ( 'NONE',  ( -15.76376720799379427, -36.50737899243800655, -17.99768973515599768 ) ) ;
#7916=LINE ( 'NONE', #13599, #9869 ) ;
#7928=EDGE_CURVE ( 'NONE', #3880, #1356, #12837, .T. ) ;
#7932=EDGE_CURVE ( 'NONE', #8709, #14890, #4913, .T. ) ;
#7936=CARTESIAN_POINT ( 'NONE',  ( -7.768926039458051491, -39.58069824233449907, -0.5710089850524957544 ) ) ;
#7940=CARTESIAN_POINT ( 'NONE',  ( -8.885174762611967481, -49.00716318639572222, 44.32840209439113721 ) ) ;
#7943=EDGE_CURVE ( 'NONE', #10539, #3880, #9652, .T. ) ;
#7953=FACE_OUTER_BOUND ( 'NONE', #4072, .T. ) ;
#7960=CARTESIAN_POINT ( 'NONE',  ( -15.49969986081099904, -27.00737899243800300, -5.497689735156002122 ) ) ;
#7977=DIRECTION ( 'NONE',  ( 1.000000000000000000, -1.291538348938060198E-32, 1.054621095516909827E-16 ) ) ;
#7983=EDGE_LOOP ( 'NONE', ( #108, #14435, #3081, #344 ) ) ;
#7987=CARTESIAN_POINT ( 'NONE',  ( -22.78937479645117392, -41.20153274115700270, -17.28248307391377736 ) ) ;
#7996=CARTESIAN_POINT ( 'NONE',  ( -7.513186133687156598, -48.97671528745461700, 19.98830884321294832 ) ) ;
#8006=CIRCLE ( 'NONE', #10697, 8.000000000000000000 ) ;
#8007=DIRECTION ( 'NONE',  ( 0.000000000000000000, -1.000000000000000000, -1.224646799147350002E-16 ) ) ;
#8014=CARTESIAN_POINT ( 'NONE',  ( -7.768926039458050603, -39.58069824233449907, 14.57562951474049129 ) ) ;
#8018=CARTESIAN_POINT ( 'NONE',  ( -15.49969986081099904, -44.50737899243799944, -109.5506571639849938 ) ) ;
#8024=DIRECTION ( 'NONE',  ( 0.000000000000000000, 0.000000000000000000, -1.000000000000000000 ) ) ;
#8058=CARTESIAN_POINT ( 'NONE',  ( -7.499699860810997265, -44.62393082527479038, 42.84690782106163454 ) ) ;
#8060=ORIENTED_EDGE ( 'NONE', *, *, #5276, .T. ) ;
#8063=EDGE_CURVE ( 'NONE', #8470, #2658, #14436, .T. ) ;
#8080=CARTESIAN_POINT ( 'NONE',  ( -7.595322498794511823, -45.75508878561614523, 46.89411779445664763 ) ) ;
#8082=AXIS2_PLACEMENT_3D ( 'NONE', #6612, #9991, #10221 ) ;
#8085=FACE_OUTER_BOUND ( 'NONE', #3596, .T. ) ;
#8094=ORIENTED_EDGE ( 'NONE', *, *, #4203, .F. ) ;
#8096=ORIENTED_EDGE ( 'NONE', *, *, #12608, .T. ) ;
#8099=VERTEX_POINT ( 'NONE', #1840 ) ;
#8112=ADVANCED_FACE ( 'NONE', ( #1763 ), #477, .F. ) ;
#8115=CARTESIAN_POINT ( 'NONE',  ( -17.58173612995575397, -52.24942676811487274, -17.94337340107023593 ) ) ;
#8117=ORIENTED_EDGE ( 'NONE', *, *, #5334, .T. ) ;
#8125=CARTESIAN_POINT ( 'NONE',  ( 3.100272115295338970, -39.60750234070978593, 52.06484617642751545 ) ) ;
#8132=AXIS2_PLACEMENT_3D ( 'NONE', #9688, #13147, #10911 ) ;
#8133=CARTESIAN_POINT ( 'NONE',  ( -7.508851067721073136, -44.91495161711613804, 21.42953195777254294 ) ) ;
#8142=ORIENTED_EDGE ( 'NONE', *, *, #5854, .F. ) ;
#8145=CARTESIAN_POINT ( 'NONE',  ( -23.48648741169278864, -43.97817952596684421, 56.14193264201148992 ) ) ;
#8147=CARTESIAN_POINT ( 'NONE',  ( -7.771455047768278668, -42.42330350419953788, -17.19278996553040528 ) ) ;
#8154=DIRECTION ( 'NONE',  ( -1.054621095516909827E-16, -1.224646799147350002E-16, 1.000000000000000000 ) ) ;
#8157=ORIENTED_EDGE ( 'NONE', *, *, #12103, .F. ) ;
#8165=ORIENTED_EDGE ( 'NONE', *, *, #11051, .T. ) ;
#8171=CARTESIAN_POINT ( 'NONE',  ( -15.49969986081098838, -17.75737899243799944, 51.00231026484400587 ) ) ;
#8175=CARTESIAN_POINT ( 'NONE',  ( -36.79886583278639023, -37.30547240248171903, 50.36646496601539980 ) ) ;
#8192=EDGE_CURVE ( 'NONE', #2509, #9604, #10246, .T. ) ;
#8194=LINE ( 'NONE', #10803, #14969 ) ;
#8196=CARTESIAN_POINT ( 'NONE',  ( 3.112640221700739840, -39.60748137431547633, -13.05276465491907345 ) ) ;
#8201=ORIENTED_EDGE ( 'NONE', *, *, #6061, .T. ) ;
#8203=ORIENTED_EDGE ( 'NONE', *, *, #1293, .T. ) ;
#8209=EDGE_CURVE ( 'NONE', #9803, #7103, #14584, .T. ) ;
#8212=CARTESIAN_POINT ( 'NONE',  ( -34.99969986081099904, -19.50737899243800300, -17.99768973515599768 ) ) ;
#8220=CARTESIAN_POINT ( 'NONE',  ( -16.54355812366951284, -36.55815850481217666, 56.99137402710550049 ) ) ;
#8223=CARTESIAN_POINT ( 'NONE',  ( -8.013558459183959926, -41.67444402531860703, -17.24300375686068421 ) ) ;
#8227=FACE_OUTER_BOUND ( 'NONE', #10327, .T. ) ;
#8237=ORIENTED_EDGE ( 'NONE', *, *, #2692, .T. ) ;
#8242=CARTESIAN_POINT ( 'NONE',  ( -5.499699860810998153, -46.50737899243799944, -8.497689735156003010 ) ) ;
#8247=CARTESIAN_POINT ( 'NONE',  ( -15.49969986081099194, -36.50737899243799944, 11.50231026484399699 ) ) ;
#8248=DIRECTION ( 'NONE',  ( 1.000000000000000000, 0.000000000000000000, 0.000000000000000000 ) ) ;
#8269=CARTESIAN_POINT ( 'NONE',  ( -7.499699860810999041, -19.50737899243799589, 54.00231026484400587 ) ) ;
#8271=CARTESIAN_POINT ( 'NONE',  ( 5.901818273210405863, -37.26927769664150958, -11.29100291904106612 ) ) ;
#8278=CARTESIAN_POINT ( 'NONE',  ( 4.144397788355465018, -38.30087877078349834, 51.44538043376633141 ) ) ;
#8286=CARTESIAN_POINT ( 'NONE',  ( -7.838594959941967311, -47.52544946159166983, -3.196372820239050228 ) ) ;
#8294=ADVANCED_FACE ( 'NONE', ( #5428 ), #13620, .F. ) ;
#8295=CARTESIAN_POINT ( 'NONE',  ( -19.04179444808664812, -37.32947002669901337, 56.83537356607605062 ) ) ;
#8305=AXIS2_PLACEMENT_3D ( 'NONE', #12342, #1559, #5226 ) ;
#8306=ORIENTED_EDGE ( 'NONE', *, *, #4402, .F. ) ;
#8319=DIRECTION ( 'NONE',  ( 0.000000000000000000, 1.850371707708594316E-16, -1.000000000000000000 ) ) ;
#8332=ADVANCED_FACE ( 'NONE', ( #3 ), #232, .F. ) ;
#8357=CARTESIAN_POINT ( 'NONE',  ( 5.737180257485530177, -37.32854632935037387, 50.40935528563701240 ) ) ;
#8359=LINE ( 'NONE', #13046, #13955 ) ;
#8363=AXIS2_PLACEMENT_3D ( 'NONE', #14467, #2770, #9944 ) ;
#8364=FACE_OUTER_BOUND ( 'NONE', #6110, .T. ) ;
#8365=CARTESIAN_POINT ( 'NONE',  ( -7.600774661674001287, -48.67202872725436436, -4.244403150344465026 ) ) ;
#8372=DIRECTION ( 'NONE',  ( -1.054621095516909827E-16, 1.224646799147350002E-16, -1.000000000000000000 ) ) ;
#8373=EDGE_LOOP ( 'NONE', ( #10035, #12622 ) ) ;
#8374=CARTESIAN_POINT ( 'NONE',  ( -9.145157332402543915, -39.61893914866874411, -17.45656333442792274 ) ) ;
#8380=CARTESIAN_POINT ( 'NONE',  ( -7.754796638793765240, -46.50763592918296752, 17.00313569000094560 ) ) ;
#8384=CIRCLE ( 'NONE', #8132, 8.000000000000000000 ) ;
#8396=MECHANICAL_DESIGN_GEOMETRIC_PRESENTATION_REPRESENTATION('',(#842),#6919);
#8400=DIRECTION ( 'NONE',  ( 0.000000000000000000, 0.000000000000000000, 1.000000000000000000 ) ) ;
#8403=CARTESIAN_POINT ( 'NONE',  ( -15.49969986081100259, -19.50737899243800300, 48.00231026484399877 ) ) ;
#8405=CARTESIAN_POINT ( 'NONE',  ( -8.559186161507744472, -48.52014164539353658, -17.35099849220764412 ) ) ;
#8408=CARTESIAN_POINT ( 'NONE',  ( -23.49969986081099194, -49.19367049345326137, -0.8113982341407305343 ) ) ;
#8422=CARTESIAN_POINT ( 'NONE',  ( -15.42469993581076970, -26.50737899243800300, 57.00223526491900117 ) ) ;
#8424=EDGE_CURVE ( 'NONE', #6799, #3424, #2123, .T. ) ;
#8427=ORIENTED_EDGE ( 'NONE', *, *, #7932, .T. ) ;
#8428=CARTESIAN_POINT ( 'NONE',  ( 6.023498351796789940, -37.22897031456926698, -11.20623205539177825 ) ) ;
#8443=PLANE ( 'NONE',  #11584 ) ;
#8446=VERTEX_POINT ( 'NONE', #10781 ) ;
#8453=ORIENTED_EDGE ( 'NONE', *, *, #7276, .T. ) ;
#8454=CARTESIAN_POINT ( 'NONE',  ( -8.313732008561206754, -40.95305761153253599, -17.30330790116151007 ) ) ;
#8460=CARTESIAN_POINT ( 'NONE',  ( -7.498776711167360887, -44.75663421272680864, 17.70716976648120422 ) ) ;
#8467=FACE_OUTER_BOUND ( 'NONE', #9519, .T. ) ;
#8470=VERTEX_POINT ( 'NONE', #5184 ) ;
#8481=CARTESIAN_POINT ( 'NONE',  ( -8.011459754790374532, -47.33491808379935861, -17.24257761966661917 ) ) ;
#8484=ORIENTED_EDGE ( 'NONE', *, *, #914, .F. ) ;
#8495=B_SPLINE_CURVE_WITH_KNOTS ( 'NONE', 3,
 ( #9692, #10844, #2809, #10916 ),
 .UNSPECIFIED., .F., .F.,
 ( 4, 4 ),
 ( 0.000000000000000000, 1.000000000000000000 ),
 .UNSPECIFIED. ) ;
#8498=CIRCLE ( 'NONE', #11925, 8.000000000000000000 ) ;
#8504=ORIENTED_EDGE ( 'NONE', *, *, #7928, .F. ) ;
#8508=EDGE_CURVE ( 'NONE', #2702, #13947, #1836, .T. ) ;
#8514=DIRECTION ( 'NONE',  ( 0.000000000000000000, 1.224646799147350002E-16, -1.000000000000000000 ) ) ;
#8519=CLOSED_SHELL ( 'NONE', ( #1680, #435, #13568, #2893, #809, #9422, #10230, #4043, #10702, #759, #13900, #13965, #13588, #1016, #12227, #8112, #10926, #4512, #458, #9456, #12296, #9148, #1141, #5045, #9510, #2012, #11493, #2252, #4645, #7267, #314, #6865, #7531, #8332, #6802, #2, #7716, #5974, #11566, #14540, #13861, #4514, #11631, #7472, #13473, #12843, #8627, #10651, #11252, #7886, #2881, #1779, #5163, #8294, #13581, #2838, #5422, #7817 ) ) ;
#8520=EDGE_LOOP ( 'NONE', ( #12997, #8993, #12499, #6223, #4828, #5161, #243, #12946, #14051, #2224, #14190, #3304, #2720, #2385, #244, #5494, #13701, #11982, #9791, #8157, #5411, #3448, #2713, #5963, #8522, #8670, #14046 ) ) ;
#8522=ORIENTED_EDGE ( 'NONE', *, *, #9723, .T. ) ;
#8525=B_SPLINE_CURVE_WITH_KNOTS ( 'NONE', 3,
 ( #13544, #3133, #12549, #7707, #12392, #5569, #4281, #10011, #10156, #13764, #992, #6560, #3290, #9013, #6709, #12624, #11244, #2139, #2066, #765, #7784, #6785, #10082, #5421, #7853, #8938 ),
 .UNSPECIFIED., .F., .F.,
 ( 4, 2, 2, 2, 2, 2, 2, 2, 2, 2, 2, 2, 4 ),
 ( 0.03783275914711289878, 0.03940993297411544971, 0.04019851988761673905, 0.04098710680111802840, 0.04177569371461931774, 0.04256428062812060015, 0.04414145445512319965, 0.04493004136862448900, 0.04571862828212578528, 0.04729580210912836397, 0.04808438902262963943, 0.04887297593613092878, 0.05045014976313349359 ),
 .UNSPECIFIED. ) ;
#8526=CARTESIAN_POINT ( 'NONE',  ( -22.68842631263146004, -48.05638050496262537, 56.30739098709261725 ) ) ;
#8536=AXIS2_PLACEMENT_3D ( 'NONE', #8923, #5405, #11299 ) ;
#8538=CARTESIAN_POINT ( 'NONE',  ( -7.532288152704643025, -45.22345379519396857, 17.35487173259670612 ) ) ;
#8543=EDGE_LOOP ( 'NONE', ( #2019, #8895 ) ) ;
#8544=DIRECTION ( 'NONE',  ( 0.000000000000000000, 0.000000000000000000, -1.000000000000000000 ) ) ;
#8546=CARTESIAN_POINT ( 'NONE',  ( -8.992083836518990125, -50.38952316532486009, 13.62016609195713812 ) ) ;
#8551=CARTESIAN_POINT ( 'NONE',  ( -7.719139325354706926, -48.17958124988508928, 17.64249027060945352 ) ) ;
#8557=CARTESIAN_POINT ( 'NONE',  ( -7.499699860810999041, -44.50737899243799944, -17.13441993860073964 ) ) ;
#8562=CARTESIAN_POINT ( 'NONE',  ( -35.09539592173130274, -38.34531428876476866, -12.47047561222863266 ) ) ;
#8573=DIRECTION ( 'NONE',  ( 0.000000000000000000, -1.000000000000000000, -1.224646799147350002E-16 ) ) ;
#8579=ORIENTED_EDGE ( 'NONE', *, *, #7276, .F. ) ;
#8587=AXIS2_PLACEMENT_3D ( 'NONE', #7432, #2701, #7654 ) ;
#8592=CARTESIAN_POINT ( 'NONE',  ( -7.516520390631882265, -48.95538363176678587, -6.022680771983879744 ) ) ;
#8610=CARTESIAN_POINT ( 'NONE',  ( -11.02548131428532940, -22.45062562374627291, 56.73443632552402249 ) ) ;
#8612=CARTESIAN_POINT ( 'NONE',  ( -7.517689378148951107, -45.05639236071581166, 17.46402815569863876 ) ) ;
#8617=( BOUNDED_CURVE ( )  B_SPLINE_CURVE ( 3, ( #213, #1507, #1434, #6006 ),
 .UNSPECIFIED., .F., .T. ) 
 B_SPLINE_CURVE_WITH_KNOTS ( ( 4, 4 ),
 ( -8.881784197001252323E-16, 1.570796326794893893 ),
 .UNSPECIFIED. ) 
 CURVE ( )  GEOMETRIC_REPRESENTATION_ITEM ( )  RATIONAL_B_SPLINE_CURVE ( ( 1.000000000000000000, 0.8047378541243654926, 0.8047378541243654926, 1.000000000000000000 ) ) 
 REPRESENTATION_ITEM ( '' )  );
#8620=CIRCLE ( 'NONE', #2025, 3.000000000000000000 ) ;
#8627=ADVANCED_FACE ( 'NONE', ( #11854 ), #14154, .F. ) ;
#8630=CARTESIAN_POINT ( 'NONE',  ( -7.795459123704175042, -47.76474896896232281, 17.34149980383660861 ) ) ;
#8637=ORIENTED_EDGE ( 'NONE', *, *, #6346, .T. ) ;
#8669=PLANE ( 'NONE',  #6001 ) ;
#8670=ORIENTED_EDGE ( 'NONE', *, *, #7943, .T. ) ;
#8680=EDGE_CURVE ( 'NONE', #2996, #2455, #7092, .T. ) ;
#8696=EDGE_CURVE ( 'NONE', #9374, #7373, #162, .T. ) ;
#8697=EDGE_CURVE ( 'NONE', #9604, #14718, #10228, .T. ) ;
#8699=CARTESIAN_POINT ( 'NONE',  ( -7.664252951136433012, -48.41696643141915501, 17.88875613834384737 ) ) ;
#8700=( BOUNDED_CURVE ( )  B_SPLINE_CURVE ( 3, ( #5178, #12223, #6239, #5331 ),
 .UNSPECIFIED., .F., .T. ) 
 B_SPLINE_CURVE_WITH_KNOTS ( ( 4, 4 ),
 ( 1.070141614390309304, 1.245066839500267530 ),
 .UNSPECIFIED. ) 
 CURVE ( )  GEOMETRIC_REPRESENTATION_ITEM ( )  RATIONAL_B_SPLINE_CURVE ( ( 1.000000000000000000, 0.9974517222217440526, 0.9974517222217440526, 1.000000000000000000 ) ) 
 REPRESENTATION_ITEM ( '' )  );
#8702=DIRECTION ( 'NONE',  ( 0.000000000000000000, 0.000000000000000000, -1.000000000000000000 ) ) ;
#8708=CARTESIAN_POINT ( 'NONE',  ( -33.91855968657274190, -40.00214821740372884, -13.16261487092677207 ) ) ;
#8709=VERTEX_POINT ( 'NONE', #5412 ) ;
#8715=DIRECTION ( 'NONE',  ( 0.000000000000000000, -1.000000000000000000, -1.224646799147350002E-16 ) ) ;
#8724=CARTESIAN_POINT ( 'NONE',  ( -15.49969986081099904, -57.00737899243801365, 57.00231026484399166 ) ) ;
#8733=AXIS2_PLACEMENT_3D ( 'NONE', #14565, #13429, #7596 ) ;
#8749=CARTESIAN_POINT ( 'NONE',  ( 2.500300139188998738, -46.50737899243799944, -2.997689735156002122 ) ) ;
#8771=AXIS2_PLACEMENT_3D ( 'NONE', #2162, #9182, #14782 ) ;
#8772=EDGE_CURVE ( 'NONE', #10639, #10198, #8779, .T. ) ;
#8779=LINE ( 'NONE', #835, #9457 ) ;
#8781=DIRECTION ( 'NONE',  ( 0.000000000000000000, 0.000000000000000000, -1.000000000000000000 ) ) ;
#8783=CARTESIAN_POINT ( 'NONE',  ( -36.73657997911097794, -37.32854632934932937, -11.40473475594660968 ) ) ;
#8787=CARTESIAN_POINT ( 'NONE',  ( -7.512805849530849400, -44.04964101872660365, -5.039951761444699585 ) ) ;
#8788=DIRECTION ( 'NONE',  ( -1.000000000000000000, -3.632077277826439854E-16, 0.000000000000000000 ) ) ;
#8796=EDGE_CURVE ( 'NONE', #14198, #10775, #12463, .T. ) ;
#8807=DIRECTION ( 'NONE',  ( 0.000000000000000000, -1.000000000000000000, -1.224646799147350002E-16 ) ) ;
#8820=CARTESIAN_POINT ( 'NONE',  ( -17.32633557924186007, -52.30049142393889383, 56.95868565438303222 ) ) ;
#8835=CIRCLE ( 'NONE', #8587, 37.50000000000000000 ) ;
#8851=CARTESIAN_POINT ( 'NONE',  ( -7.886584594865190034, -46.96511696614950182, -7.955427708867500058 ) ) ;
#8855=CARTESIAN_POINT ( 'NONE',  ( -7.507568439312231057, -44.88869056754154485, -3.592341908997338074 ) ) ;
#8857=ORIENTED_EDGE ( 'NONE', *, *, #7360, .F. ) ;
#8867=CARTESIAN_POINT ( 'NONE',  ( -3.499699860810999041, -57.00737899243800655, 55.03046811182510112 ) ) ;
#8870=DIRECTION ( 'NONE',  ( 0.000000000000000000, 0.000000000000000000, 1.000000000000000000 ) ) ;
#8875=ORIENTED_EDGE ( 'NONE', *, *, #12567, .T. ) ;
#8876=CARTESIAN_POINT ( 'NONE',  ( 7.500300139189000070, -37.00737899243799944, 49.12071670408379731 ) ) ;
#8888=EDGE_CURVE ( 'NONE', #1356, #7229, #14135, .T. ) ;
#8890=PLANE ( 'NONE',  #8305 ) ;
#8895=ORIENTED_EDGE ( 'NONE', *, *, #13359, .T. ) ;
#8910=DIRECTION ( 'NONE',  ( -1.000000000000000000, 1.291538348938060198E-32, -1.054621095516909827E-16 ) ) ;
#8911=ORIENTED_EDGE ( 'NONE', *, *, #12432, .T. ) ;
#8918=DIRECTION ( 'NONE',  ( 1.054621095516909827E-16, 0.000000000000000000, -1.000000000000000000 ) ) ;
#8923=CARTESIAN_POINT ( 'NONE',  ( 2.500300139188996518, -46.50737899243799944, 44.50231026484399877 ) ) ;
#8938=CARTESIAN_POINT ( 'NONE',  ( -15.49969986081099904, -52.50737899243799944, 57.00231026484399166 ) ) ;
#8939=DIRECTION ( 'NONE',  ( 0.000000000000000000, 1.000000000000000000, 1.224646799147350002E-16 ) ) ;
#8941=AXIS2_PLACEMENT_3D ( 'NONE', #12326, #1843, #6488 ) ;
#8947=LINE ( 'NONE', #10167, #10799 ) ;
#8952=CARTESIAN_POINT ( 'NONE',  ( -7.886584594865190034, -46.96511696614940234, 17.04457229113261718 ) ) ;
#8953=CARTESIAN_POINT ( 'NONE',  ( -7.499699860810999041, -19.50737899243799589, 48.00231026484399877 ) ) ;
#8966=EDGE_CURVE ( 'NONE', #10775, #11940, #7131, .T. ) ;
#8973=CARTESIAN_POINT ( 'NONE',  ( -11.02342383152550553, -36.50737899243796392, 27.50231026484403074 ) ) ;
#8978=VECTOR ( 'NONE', #2939, 1000.000000000000000 ) ;
#8984=DIRECTION ( 'NONE',  ( 0.000000000000000000, -1.000000000000000000, -1.224646799147350002E-16 ) ) ;
#8988=VERTEX_POINT ( 'NONE', #14288 ) ;
#8989=DIRECTION ( 'NONE',  ( 0.000000000000000000, 0.000000000000000000, -1.000000000000000000 ) ) ;
#8991=CARTESIAN_POINT ( 'NONE',  ( -17.57474910601409235, -36.77673389236314705, -17.94107779625593579 ) ) ;
#8993=ORIENTED_EDGE ( 'NONE', *, *, #8192, .T. ) ;
#9002=CARTESIAN_POINT ( 'NONE',  ( -15.49969986081099904, -57.00737899243801365, 57.00231026484399166 ) ) ;
#9005=CARTESIAN_POINT ( 'NONE',  ( -7.508969231007553091, -44.91770256118098104, -3.568200169185395065 ) ) ;
#9013=CARTESIAN_POINT ( 'NONE',  ( -10.02412658163347636, -50.34568278964318466, 56.60086416076374860 ) ) ;
#9027=ORIENTED_EDGE ( 'NONE', *, *, #6043, .T. ) ;
#9028=B_SPLINE_CURVE_WITH_KNOTS ( 'NONE', 3,
 ( #14188, #11814, #9748, #1339, #2482, #3632 ),
 .UNSPECIFIED., .F., .F.,
 ( 4, 2, 4 ),
 ( 0.7879834095039132125, 0.8939917047519565507, 1.000000000000000000 ),
 .UNSPECIFIED. ) ;
#9039=CARTESIAN_POINT ( 'NONE',  ( -7.879287384819335216, -47.08648443922195526, -7.932823793481322383 ) ) ;
#9043=VERTEX_POINT ( 'NONE', #4103 ) ;
#9047=CARTESIAN_POINT ( 'NONE',  ( 2.581287997393676203, -41.10853556844468670, 52.35544040764929719 ) ) ;
#9049=CARTESIAN_POINT ( 'NONE',  ( -15.49969986081099016, -36.50737899243799944, 27.50231026484399521 ) ) ;
#9056=CARTESIAN_POINT ( 'NONE',  ( -7.503607783881640181, -44.63988287651423548, 21.17968396569539280 ) ) ;
#9060=ORIENTED_EDGE ( 'NONE', *, *, #5297, .T. ) ;
#9067=CARTESIAN_POINT ( 'NONE',  ( -21.52722649236416430, -39.22145586813481088, -17.51198461415464180 ) ) ;
#9085=CARTESIAN_POINT ( 'NONE',  ( -7.499699860810999930, -44.62460413890913458, 46.15861046013883140 ) ) ;
#9088=CARTESIAN_POINT ( 'NONE',  ( -0.3742611254310274083, -27.95036676736705417, -14.90232471354687860 ) ) ;
#9092=CARTESIAN_POINT ( 'NONE',  ( -8.708182160528487259, -48.73602156695860543, 43.35738220827035860 ) ) ;
#9098=DIRECTION ( 'NONE',  ( -0.8660254037844387076, -0.4999999999999998890, 0.000000000000000000 ) ) ;
#9113=( NAMED_UNIT ( * ) PLANE_ANGLE_UNIT ( ) SI_UNIT ( $, .RADIAN. ) );
#9117=CARTESIAN_POINT ( 'NONE',  ( -23.43509953878110608, -45.55571247603148066, -17.14847601522437870 ) ) ;
#9122=ORIENTED_EDGE ( 'NONE', *, *, #9612, .F. ) ;
#9134=ORIENTED_EDGE ( 'NONE', *, *, #3434, .F. ) ;
#9140=EDGE_CURVE ( 'NONE', #5678, #5628, #5544, .T. ) ;
#9148=ADVANCED_FACE ( 'NONE', ( #14583 ), #6380, .T. ) ;
#9156=AXIS2_PLACEMENT_3D ( 'NONE', #2593, #11923, #2668 ) ;
#9167=CARTESIAN_POINT ( 'NONE',  ( -7.753733168396166775, -46.50737899243799944, 42.00231026484399166 ) ) ;
#9168=CARTESIAN_POINT ( 'NONE',  ( -15.49969986081099371, -57.00737899243799944, -17.99768973515599768 ) ) ;
#9176=DIRECTION ( 'NONE',  ( 0.000000000000000000, -1.000000000000000000, -1.224646799147350002E-16 ) ) ;
#9178=ORIENTED_EDGE ( 'NONE', *, *, #8508, .F. ) ;
#9182=DIRECTION ( 'NONE',  ( -0.8660254037844387076, 0.4999999999999998890, 0.000000000000000000 ) ) ;
#9184=( NAMED_UNIT ( * ) SI_UNIT ( $, .STERADIAN. ) SOLID_ANGLE_UNIT ( ) );
#9187=CARTESIAN_POINT ( 'NONE',  ( -18.80870833456381419, -51.79568668368815310, -17.85220341531665156 ) ) ;
#9194=ORIENTED_EDGE ( 'NONE', *, *, #5690, .F. ) ;
#9202=EDGE_CURVE ( 'NONE', #8470, #5287, #6548, .T. ) ;
#9203=CARTESIAN_POINT ( 'NONE',  ( -7.509245100188403299, -44.92199632866380909, 21.43533231848149967 ) ) ;
#9216=ORIENTED_EDGE ( 'NONE', *, *, #10868, .F. ) ;
#9231=CARTESIAN_POINT ( 'NONE',  ( -5.499699860811004370, -46.50737899243799944, 47.00231026484399877 ) ) ;
#9238=LINE ( 'NONE', #74, #64 ) ;
#9239=CARTESIAN_POINT ( 'NONE',  ( -15.49969986081099904, -32.00737899243799944, 19.50231026484400232 ) ) ;
#9246=DIRECTION ( 'NONE',  ( 1.000000000000000000, 0.000000000000000000, 0.000000000000000000 ) ) ;
#9247=EDGE_CURVE ( 'NONE', #9646, #6722, #9728, .T. ) ;
#9257=EDGE_CURVE ( 'NONE', #11105, #3128, #8498, .T. ) ;
#9270=CARTESIAN_POINT ( 'NONE',  ( -20.37445634772518233, -50.85598640664056802, -17.68005340029201022 ) ) ;
#9273=ORIENTED_EDGE ( 'NONE', *, *, #8772, .T. ) ;
#9287=PLANE ( 'NONE',  #10724 ) ;
#9288=ORIENTED_EDGE ( 'NONE', *, *, #1602, .T. ) ;
#9290=LINE ( 'NONE', #10519, #11812 ) ;
#9295=CARTESIAN_POINT ( 'NONE',  ( -23.49969986081100259, -44.50737899243799944, 56.13904046828872652 ) ) ;
#9296=ORIENTED_EDGE ( 'NONE', *, *, #6896, .F. ) ;
#9300=EDGE_CURVE ( 'NONE', #6631, #10198, #5271, .T. ) ;
#9302=CARTESIAN_POINT ( 'NONE',  ( 2.500300139188999182, -42.00737899243800655, 19.50231026484398811 ) ) ;
#9309=EDGE_LOOP ( 'NONE', ( #2860, #4712 ) ) ;
#9315=CARTESIAN_POINT ( 'NONE',  ( -7.495514965259227225, -43.99345095228513003, 19.65834624315599299 ) ) ;
#9318=DIRECTION ( 'NONE',  ( -1.734723475976808080E-16, 0.000000000000000000, 1.000000000000000000 ) ) ;
#9319=CARTESIAN_POINT ( 'NONE',  ( -8.123614162940384631, -47.60880580837400800, 46.75233648801069819 ) ) ;
#9321=AXIS2_PLACEMENT_3D ( 'NONE', #4718, #14351, #9526 ) ;
#9323=CARTESIAN_POINT ( 'NONE',  ( -15.49969986081100259, -19.50737899243800300, 51.00231026484400587 ) ) ;
#9324=CARTESIAN_POINT ( 'NONE',  ( -7.752363797594655992, -48.01475789269080252, -7.497332716824399057 ) ) ;
#9325=CARTESIAN_POINT ( 'NONE',  ( -36.84926662630419969, -37.28744580235390771, 50.33162166081972089 ) ) ;
#9329=VERTEX_POINT ( 'NONE', #3636 ) ;
#9337=ORIENTED_EDGE ( 'NONE', *, *, #4232, .T. ) ;
#9338=VECTOR ( 'NONE', #728, 1000.000000000000000 ) ;
#9339=VECTOR ( 'NONE', #13964, 1000.000000000000000 ) ;
#9342=EDGE_CURVE ( 'NONE', #12721, #3694, #11660, .T. ) ;
#9352=CARTESIAN_POINT ( 'NONE',  ( 6.481863649926076221, -37.10904096101434391, -10.88012559947874891 ) ) ;
#9355=ORIENTED_EDGE ( 'NONE', *, *, #13810, .T. ) ;
#9365=CARTESIAN_POINT ( 'NONE',  ( -15.49969986081099904, -36.50737899243799944, -13.49768973515600479 ) ) ;
#9374=VERTEX_POINT ( 'NONE', #1493 ) ;
#9378=CARTESIAN_POINT ( 'NONE',  ( -17.58100468212644429, -36.76477499413114458, 56.94810725308578014 ) ) ;
#9390=EDGE_LOOP ( 'NONE', ( #6666, #14999, #12756, #7022, #12056, #8094 ) ) ;
#9391=CARTESIAN_POINT ( 'NONE',  ( -2.716578225681299141, -32.00737899243799944, 54.75627176226269199 ) ) ;
#9400=DIRECTION ( 'NONE',  ( 0.000000000000000000, 0.000000000000000000, 1.000000000000000000 ) ) ;
#9406=CARTESIAN_POINT ( 'NONE',  ( -7.799975386333926508, -47.73689692355252134, -7.674474215535603605 ) ) ;
#9419=CARTESIAN_POINT ( 'NONE',  ( 2.500300139188999182, -37.00737899243799944, -13.39525803434800011 ) ) ;
#9422=ADVANCED_FACE ( 'NONE', ( #9598 ), #4713, .F. ) ;
#9427=CARTESIAN_POINT ( 'NONE',  ( 2.708095644062286311, -40.57968410433875306, -13.28071779296938004 ) ) ;
#9433=CARTESIAN_POINT ( 'NONE',  ( 2.919159964955403197, -40.00214821739496074, 52.16723540061214237 ) ) ;
#9436=CARTESIAN_POINT ( 'NONE',  ( -15.49969986081099904, -27.00737899243800300, 19.50231026484400587 ) ) ;
#9442=CARTESIAN_POINT ( 'NONE',  ( -7.886584594865180264, -46.96511696614940234, -3.039951761444701361 ) ) ;
#9443=DIRECTION ( 'NONE',  ( 1.054621095516909827E-16, -1.224646799147350002E-16, 1.000000000000000000 ) ) ;
#9449=LINE ( 'NONE', #14122, #2745 ) ;
#9456=ADVANCED_FACE ( 'NONE', ( #5380 ), #4081, .T. ) ;
#9457=VECTOR ( 'NONE', #12383, 1000.000000000000000 ) ;
#9474=EDGE_CURVE ( 'NONE', #1679, #7202, #5235, .T. ) ;
#9481=CARTESIAN_POINT ( 'NONE',  ( -13.42276483944220189, -52.23752306156875136, -17.94097413569642185 ) ) ;
#9483=CARTESIAN_POINT ( 'NONE',  ( -35.79116231783276447, -37.80121036461405026, 51.03851805053808732 ) ) ;
#9504=ORIENTED_EDGE ( 'NONE', *, *, #1013, .F. ) ;
#9505=EDGE_LOOP ( 'NONE', ( #7043, #4777 ) ) ;
#9510=ADVANCED_FACE ( 'NONE', ( #13282 ), #2789, .F. ) ;
#9517=CARTESIAN_POINT ( 'NONE',  ( -7.501378586840250939, -49.00244658604244563, -5.658025522608453706 ) ) ;
#9519=EDGE_LOOP ( 'NONE', ( #11312, #12164, #14622, #4888 ) ) ;
#9526=DIRECTION ( 'NONE',  ( 1.054621095516909827E-16, 0.000000000000000000, -1.000000000000000000 ) ) ;
#9535=CARTESIAN_POINT ( 'NONE',  ( -7.661865618943386913, -46.13483245617170780, 17.00230869392893496 ) ) ;
#9539=CARTESIAN_POINT ( 'NONE',  ( 1.872105016583413661, -24.05954647699556048, 52.82914930240929863 ) ) ;
#9547=CARTESIAN_POINT ( 'NONE',  ( -7.754798889200088752, -46.50763646577239285, -7.996864293225370623 ) ) ;
#9549=CARTESIAN_POINT ( 'NONE',  ( -15.49969986081099904, -27.00737899243800300, -5.497689735156002122 ) ) ;
#9553=CARTESIAN_POINT ( 'NONE',  ( 2.500300139188999182, -37.00737899243799944, 52.39987856403599409 ) ) ;
#9555=CARTESIAN_POINT ( 'NONE',  ( -14.97606084353312639, -52.50737899243799234, -17.99768973515599413 ) ) ;
#9556=CARTESIAN_POINT ( 'NONE',  ( -33.70749536570576765, -40.57968410429901951, 52.28533832264545822 ) ) ;
#9567=VERTEX_POINT ( 'NONE', #5153 ) ;
#9570=VECTOR ( 'NONE', #13408, 1000.000000000000000 ) ;
#9574=EDGE_CURVE ( 'NONE', #2509, #1356, #5804, .T. ) ;
#9579=ORIENTED_EDGE ( 'NONE', *, *, #7572, .T. ) ;
#9585=CARTESIAN_POINT ( 'NONE',  ( 5.263246529796798079, -37.53054613522389360, 50.73053146564911486 ) ) ;
#9589=CARTESIAN_POINT ( 'NONE',  ( -7.768926039458054156, -39.58069824233449907, -10.42437048525951404 ) ) ;
#9594=EDGE_CURVE ( 'NONE', #12480, #9329, #4607, .T. ) ;
#9598=FACE_OUTER_BOUND ( 'NONE', #5456, .T. ) ;
#9601=ORIENTED_EDGE ( 'NONE', *, *, #13012, .F. ) ;
#9603=CARTESIAN_POINT ( 'NONE',  ( -21.52375782506408086, -39.21750366204430804, 56.51717219687775184 ) ) ;
#9604=VERTEX_POINT ( 'NONE', #6220 ) ;
#9605=CARTESIAN_POINT ( 'NONE',  ( -9.477415257007141491, -39.21568696007443577, -17.51282566149688336 ) ) ;
#9612=EDGE_CURVE ( 'NONE', #1229, #7911, #13575, .T. ) ;
#9618=EDGE_CURVE ( 'NONE', #10750, #11940, #4311, .T. ) ;
#9630=DIRECTION ( 'NONE',  ( 0.000000000000000000, -1.000000000000000000, -1.224646799147350002E-16 ) ) ;
#9634=ORIENTED_EDGE ( 'NONE', *, *, #8680, .F. ) ;
#9637=CARTESIAN_POINT ( 'NONE',  ( -33.65972808787644510, -40.75169664996035834, 52.31182291862857880 ) ) ;
#9641=ORIENTED_EDGE ( 'NONE', *, *, #8680, .T. ) ;
#9646=VERTEX_POINT ( 'NONE', #6583 ) ;
#9652=LINE ( 'NONE', #9419, #13458 ) ;
#9658=CARTESIAN_POINT ( 'NONE',  ( -27.49969986081100259, -57.00737899243800655, 55.03046811182510112 ) ) ;
#9659=VERTEX_POINT ( 'NONE', #871 ) ;
#9662=ORIENTED_EDGE ( 'NONE', *, *, #16, .F. ) ;
#9670=VECTOR ( 'NONE', #13976, 1000.000000000000000 ) ;
#9679=DIRECTION ( 'NONE',  ( 0.000000000000000000, -1.000000000000000000, -1.224646799147350002E-16 ) ) ;
#9683=VECTOR ( 'NONE', #5283, 1000.000000000000000 ) ;
#9686=CARTESIAN_POINT ( 'NONE',  ( -10.99662508417897477, -22.43611682583629019, 56.73095874158131124 ) ) ;
#9688=CARTESIAN_POINT ( 'NONE',  ( -15.49969986081099194, -27.00737899243800300, 19.50231026484399877 ) ) ;
#9692=CARTESIAN_POINT ( 'NONE',  ( -7.512805849530849400, -44.04964101872660365, -5.039951761444699585 ) ) ;
#9695=CARTESIAN_POINT ( 'NONE',  ( -15.42469986081099442, -23.50709773848280904, 54.00231026484400587 ) ) ;
#9697=ORIENTED_EDGE ( 'NONE', *, *, #8888, .T. ) ;
#9698=VECTOR ( 'NONE', #6720, 1000.000000000000000 ) ;
#9699=DIRECTION ( 'NONE',  ( 0.000000000000000000, 0.000000000000000000, 1.000000000000000000 ) ) ;
#9702=CARTESIAN_POINT ( 'NONE',  ( 4.000300139189000959, -20.37340439622241917, -12.52892449124999885 ) ) ;
#9710=CARTESIAN_POINT ( 'NONE',  ( -7.499699860810999041, -44.50737899243799944, -109.5506571639849938 ) ) ;
#9713=CARTESIAN_POINT ( 'NONE',  ( -7.504568435050878783, -44.41879534613468650, -4.116207154834379267 ) ) ;
#9716=CARTESIAN_POINT ( 'NONE',  ( -33.55125091640665147, -41.28719780951828966, -13.36700348819730699 ) ) ;
#9723=EDGE_CURVE ( 'NONE', #14455, #10539, #1615, .T. ) ;
#9728=CIRCLE ( 'NONE', #14115, 2.999999999999999112 ) ;
#9729=CARTESIAN_POINT ( 'NONE',  ( -27.49969986081100259, -57.00737899243800655, -16.02584758213710003 ) ) ;
#9748=CARTESIAN_POINT ( 'NONE',  ( -7.505482346041832287, -44.32791517324671560, 20.74177506415496453 ) ) ;
#9754=EDGE_LOOP ( 'NONE', ( #6497, #9811, #9504, #8484, #2902 ) ) ;
#9757=EDGE_CURVE ( 'NONE', #4806, #6735, #5070, .T. ) ;
#9759=ORIENTED_EDGE ( 'NONE', *, *, #8888, .F. ) ;
#9766=CYLINDRICAL_SURFACE ( 'NONE', #6178, 8.000000000000000000 ) ;
#9773=FACE_OUTER_BOUND ( 'NONE', #8373, .T. ) ;
#9776=DIRECTION ( 'NONE',  ( -1.000000000000000000, 1.291538348938060198E-32, -1.054621095516909827E-16 ) ) ;
#9781=DIRECTION ( 'NONE',  ( 0.000000000000000000, 0.000000000000000000, -1.000000000000000000 ) ) ;
#9791=ORIENTED_EDGE ( 'NONE', *, *, #9892, .F. ) ;
#9801=CARTESIAN_POINT ( 'NONE',  ( -7.510314868261046328, -44.09321551920025684, 45.16549881609444128 ) ) ;
#9803=VERTEX_POINT ( 'NONE', #1848 ) ;
#9806=CARTESIAN_POINT ( 'NONE',  ( 2.500300139188999182, -51.00737899243799944, 52.39987856403599409 ) ) ;
#9807=ORIENTED_EDGE ( 'NONE', *, *, #1414, .T. ) ;
#9811=ORIENTED_EDGE ( 'NONE', *, *, #5048, .T. ) ;
#9830=CARTESIAN_POINT ( 'NONE',  ( -22.44301654231075815, -48.51543857339960653, 56.35509430644546569 ) ) ;
#9839=CARTESIAN_POINT ( 'NONE',  ( -11.06590827715117520, -22.47078556645032066, 56.73927296486425575 ) ) ;
#9840=CARTESIAN_POINT ( 'NONE',  ( -23.49969986081100615, -39.82108749142274462, 14.81601876382873506 ) ) ;
#9844=EDGE_CURVE ( 'NONE', #1516, #9043, #6349, .T. ) ;
#9851=CARTESIAN_POINT ( 'NONE',  ( -23.49969986081099904, -44.50737899243799944, -109.5506571639849938 ) ) ;
#9852=ORIENTED_EDGE ( 'NONE', *, *, #9474, .F. ) ;
#9857=CARTESIAN_POINT ( 'NONE',  ( -7.886584594865190034, -46.96511696614940234, 17.04457229113261718 ) ) ;
#9858=AXIS2_PLACEMENT_3D ( 'NONE', #5251, #734, #2031 ) ;
#9866=CARTESIAN_POINT ( 'NONE',  ( -36.05468215437335289, -37.64246294775075796, -11.86277418255565053 ) ) ;
#9868=ORIENTED_EDGE ( 'NONE', *, *, #2780, .T. ) ;
#9869=VECTOR ( 'NONE', #2043, 1000.000000000000000 ) ;
#9875=EDGE_CURVE ( 'NONE', #6512, #6717, #4065, .T. ) ;
#9882=CARTESIAN_POINT ( 'NONE',  ( 0.5796456139481083181, -52.92803351767888387, 53.45077026338344695 ) ) ;
#9892=EDGE_CURVE ( 'NONE', #13194, #12587, #7646, .T. ) ;
#9898=ORIENTED_EDGE ( 'NONE', *, *, #5870, .F. ) ;
#9900=EDGE_LOOP ( 'NONE', ( #1791, #2174 ) ) ;
#9903=VERTEX_POINT ( 'NONE', #8876 ) ;
#9922=CARTESIAN_POINT ( 'NONE',  ( -7.799975386333939831, -47.73689692355232239, 17.32552578446427560 ) ) ;
#9923=EDGE_CURVE ( 'NONE', #2754, #1528, #8947, .T. ) ;
#9928=CARTESIAN_POINT ( 'NONE',  ( -7.705994742804308295, -46.29709259384130604, -3.005990668410089217 ) ) ;
#9936=FACE_OUTER_BOUND ( 'NONE', #8520, .T. ) ;
#9944=DIRECTION ( 'NONE',  ( -1.291538348938060198E-32, 1.000000000000000000, 0.000000000000000000 ) ) ;
#9966=CIRCLE ( 'NONE', #10206, 10.00000000000000000 ) ;
#9991=DIRECTION ( 'NONE',  ( 0.000000000000000000, -1.000000000000000000, -1.224646799147350002E-16 ) ) ;
#9995=AXIS2_PLACEMENT_3D ( 'NONE', #2005, #861, #4453 ) ;
#10007=DIRECTION ( 'NONE',  ( -1.000000000000000000, 1.291538348938060198E-32, -1.054621095516909827E-16 ) ) ;
#10011=CARTESIAN_POINT ( 'NONE',  ( -8.209920852191324059, -47.81297650378272834, 56.28708271300973109 ) ) ;
#10013=DIRECTION ( 'NONE',  ( 0.000000000000000000, 1.224646799147350002E-16, -1.000000000000000000 ) ) ;
#10016=CYLINDRICAL_SURFACE ( 'NONE', #14815, 8.000000000000000000 ) ;
#10017=CARTESIAN_POINT ( 'NONE',  ( -7.512805849530849400, -44.04964101872660365, 19.96004823855532706 ) ) ;
#10020=VERTEX_POINT ( 'NONE', #4672 ) ;
#10021=LINE ( 'NONE', #6495, #2179 ) ;
#10033=CARTESIAN_POINT ( 'NONE',  ( 4.000300139189000959, -20.37340439622242982, 51.53354502093799994 ) ) ;
#10035=ORIENTED_EDGE ( 'NONE', *, *, #1537, .T. ) ;
#10041=CARTESIAN_POINT ( 'NONE',  ( 2.500300139188999182, -46.50737899243799944, 19.50231026484399877 ) ) ;
#10051=FACE_OUTER_BOUND ( 'NONE', #199, .T. ) ;
#10058=CIRCLE ( 'NONE', #11785, 8.000000000000000000 ) ;
#10059=DIRECTION ( 'NONE',  ( 1.000000000000000000, -1.291538348938060198E-32, 1.054621095516909827E-16 ) ) ;
#10068=CARTESIAN_POINT ( 'NONE',  ( -7.570456978157269035, -48.78587553029987589, 20.54355782397079722 ) ) ;
#10072=CARTESIAN_POINT ( 'NONE',  ( -15.57469986081099478, -23.50737899243800300, 56.85231026484400019 ) ) ;
#10078=CARTESIAN_POINT ( 'NONE',  ( -33.70353523260111928, -40.58388572172528086, -13.28296881874997126 ) ) ;
#10082=CARTESIAN_POINT ( 'NONE',  ( -13.67949125328055793, -52.30193472759165729, 56.95898663485335334 ) ) ;
#10085=DIRECTION ( 'NONE',  ( 0.000000000000000000, 1.224646799147350002E-16, -1.000000000000000000 ) ) ;
#10091=DIRECTION ( 'NONE',  ( 1.445602896647339656E-16, 0.000000000000000000, -1.000000000000000000 ) ) ;
#10094=DIRECTION ( 'NONE',  ( 0.000000000000000000, 1.000000000000000000, 1.224646799147350002E-16 ) ) ;
#10102=B_SPLINE_CURVE_WITH_KNOTS ( 'NONE', 3,
 ( #5724, #9315, #11616, #1132 ),
 .UNSPECIFIED., .F., .F.,
 ( 4, 4 ),
 ( 0.000000000000000000, 1.000000000000000000 ),
 .UNSPECIFIED. ) ;
#10112=CARTESIAN_POINT ( 'NONE',  ( -15.42470001081054498, -57.00737899243800655, 57.00223526506900384 ) ) ;
#10120=CARTESIAN_POINT ( 'NONE',  ( -9.481988904325579171, -39.22957468916221302, 56.51670373693783489 ) ) ;
#10124=VECTOR ( 'NONE', #14837, 1000.000000000000000 ) ;
#10136=CARTESIAN_POINT ( 'NONE',  ( -15.49969986081099727, -27.00737899243800300, 2.502310264843997878 ) ) ;
#10149=CARTESIAN_POINT ( 'NONE',  ( -5.499699860811003482, -46.50737899243799944, 44.50231026484399877 ) ) ;
#10156=CARTESIAN_POINT ( 'NONE',  ( -8.321349321884236261, -48.04850127655814873, 56.30906253082663682 ) ) ;
#10166=ORIENTED_EDGE ( 'NONE', *, *, #11051, .F. ) ;
#10167=CARTESIAN_POINT ( 'NONE',  ( -15.57469986081099478, -23.50709773848280904, 54.00231026484400587 ) ) ;
#10182=DIRECTION ( 'NONE',  ( 0.000000000000000000, 0.000000000000000000, -1.000000000000000000 ) ) ;
#10192=DIRECTION ( 'NONE',  ( 1.445602896647337931E-16, 0.000000000000000000, -1.000000000000000000 ) ) ;
#10195=CARTESIAN_POINT ( 'NONE',  ( 2.500300139188996518, -41.82625798755428548, 52.39987856403597988 ) ) ;
#10197=EDGE_CURVE ( 'NONE', #9374, #12241, #2129, .T. ) ;
#10198=VERTEX_POINT ( 'NONE', #7333 ) ;
#10206=AXIS2_PLACEMENT_3D ( 'NONE', #1921, #6792, #14772 ) ;
#10208=CARTESIAN_POINT ( 'NONE',  ( 2.500300139188999182, -46.50737899243799944, -5.497689735156002122 ) ) ;
#10210=LINE ( 'NONE', #4553, #3130 ) ;
#10214=ORIENTED_EDGE ( 'NONE', *, *, #11305, .T. ) ;
#10217=CARTESIAN_POINT ( 'NONE',  ( -15.49969986081099727, -52.50737899243799944, 2.502310264843994769 ) ) ;
#10221=DIRECTION ( 'NONE',  ( 0.000000000000000000, 0.000000000000000000, -1.000000000000000000 ) ) ;
#10226=CARTESIAN_POINT ( 'NONE',  ( -7.629407442448590260, -48.55937836028767407, 20.93097002895218495 ) ) ;
#10228=B_SPLINE_CURVE_WITH_KNOTS ( 'NONE', 3,
 ( #12010, #9555, #6251, #13018, #9481, #14450, #4824, #6181, #14231, #10933, #3748, #10863, #13242, #3674, #12943, #14306, #2523, #8405, #1452, #8481, #390, #5050, #5121, #14382, #3898, #8557 ),
 .UNSPECIFIED., .F., .F.,
 ( 4, 2, 2, 2, 2, 2, 2, 2, 2, 2, 2, 2, 4 ),
 ( 0.03783278222213234954, 0.03940995139284290266, 0.04019853597819818269, 0.04098712056355345579, 0.04177570514890873582, 0.04256428973426400891, 0.04414145890497456204, 0.04493004349032983513, 0.04571862807568510823, 0.04729579724639566135, 0.04808438183175094138, 0.04887296641710622142, 0.05045013558781678148 ),
 .UNSPECIFIED. ) ;
#10230=ADVANCED_FACE ( 'NONE', ( #10444 ), #5770, .F. ) ;
#10237=EDGE_LOOP ( 'NONE', ( #12494, #6472, #10824, #11273, #13857 ) ) ;
#10238=CARTESIAN_POINT ( 'NONE',  ( -7.517316220913920155, -45.05891496665708473, 46.54929868018043493 ) ) ;
#10244=CARTESIAN_POINT ( 'NONE',  ( 2.500300139188999182, -46.50737899243799944, 19.50231026484399877 ) ) ;
#10246=LINE ( 'NONE', #9168, #4816 ) ;
#10251=FACE_OUTER_BOUND ( 'NONE', #1081, .T. ) ;
#10252=EDGE_LOOP ( 'NONE', ( #9296, #3164, #14367, #2022, #3540, #5416, #13782, #661 ) ) ;
#10266=( BOUNDED_CURVE ( )  B_SPLINE_CURVE ( 3, ( #10460, #4727, #2357, #14056 ),
 .UNSPECIFIED., .F., .T. ) 
 B_SPLINE_CURVE_WITH_KNOTS ( ( 4, 4 ),
 ( 3.141592653589793116, 4.712388980384689674 ),
 .UNSPECIFIED. ) 
 CURVE ( )  GEOMETRIC_REPRESENTATION_ITEM ( )  RATIONAL_B_SPLINE_CURVE ( ( 1.000000000000000000, 0.8047378541243649375, 0.8047378541243649375, 1.000000000000000000 ) ) 
 REPRESENTATION_ITEM ( '' )  );
#10267=EDGE_LOOP ( 'NONE', ( #4431, #12256, #12575, #11499 ) ) ;
#10268=CARTESIAN_POINT ( 'NONE',  ( -19.73323262537018508, -51.30037923254471366, -17.75858867747328418 ) ) ;
#10270=ORIENTED_EDGE ( 'NONE', *, *, #12152, .T. ) ;
#10274=ORIENTED_EDGE ( 'NONE', *, *, #9844, .T. ) ;
#10279=CARTESIAN_POINT ( 'NONE',  ( -8.324915140515775747, -40.95899558977754396, 56.30975957592992387 ) ) ;
#10282=EDGE_CURVE ( 'NONE', #11225, #569, #3335, .T. ) ;
#10286=PLANE ( 'NONE',  #11937 ) ;
#10288=DIRECTION ( 'NONE',  ( 0.000000000000000000, 0.000000000000000000, -1.000000000000000000 ) ) ;
#10290=VERTEX_POINT ( 'NONE', #4413 ) ;
#10293=CARTESIAN_POINT ( 'NONE',  ( -21.85724566142533121, -39.62315458006131053, -17.45603278757056387 ) ) ;
#10294=CARTESIAN_POINT ( 'NONE',  ( -5.499699860810997265, -46.50737899243799944, -7.997689735156003010 ) ) ;
#10306=ORIENTED_EDGE ( 'NONE', *, *, #14539, .F. ) ;
#10319=DIRECTION ( 'NONE',  ( 0.000000000000000000, -1.850371707708594563E-16, 1.000000000000000000 ) ) ;
#10320=CARTESIAN_POINT ( 'NONE',  ( -8.885611223908250977, -49.00780472460828463, 44.84073519055883139 ) ) ;
#10325=CARTESIAN_POINT ( 'NONE',  ( -36.81467648506759360, -37.29975643136121022, 50.35554694645792040 ) ) ;
#10326=DIRECTION ( 'NONE',  ( 1.000000000000000000, -1.291538348938060198E-32, 1.054621095516909827E-16 ) ) ;
#10327=EDGE_LOOP ( 'NONE', ( #6315, #14630, #4262, #624, #1362, #7635, #9807, #8060, #8096, #9898, #13241, #14528, #8117, #888, #14699, #7828, #14259, #8142, #6259, #4149, #8427, #13959, #9355, #3184, #14776, #9060, #10214 ) ) ;
#10331=ORIENTED_EDGE ( 'NONE', *, *, #214, .F. ) ;
#10339=( LENGTH_UNIT ( ) NAMED_UNIT ( * ) SI_UNIT ( .MILLI., .METRE. ) );
#10344=CARTESIAN_POINT ( 'NONE',  ( -20.77774051523950050, -50.52488293980518108, -17.62495337501153259 ) ) ;
#10348=CARTESIAN_POINT ( 'NONE',  ( -15.49969986081100082, -19.50737899243800300, 19.50231026484399877 ) ) ;
#10354=CARTESIAN_POINT ( 'NONE',  ( -23.04246617642294837, -20.11702390495540982, 56.23888206045033655 ) ) ;
#10355=AXIS2_PLACEMENT_3D ( 'NONE', #2396, #7477, #14448 ) ;
#10366=CARTESIAN_POINT ( 'NONE',  ( -15.49969986081099904, -37.00737899243799944, 19.50231026484400232 ) ) ;
#10368=ORIENTED_EDGE ( 'NONE', *, *, #2556, .T. ) ;
#10370=CARTESIAN_POINT ( 'NONE',  ( -16.55105184719503697, -36.57242519587391172, -17.98385852237137428 ) ) ;
#10374=EDGE_CURVE ( 'NONE', #8446, #12112, #10673, .T. ) ;
#10386=DIRECTION ( 'NONE',  ( 0.000000000000000000, 0.000000000000000000, -1.000000000000000000 ) ) ;
#10389=ORIENTED_EDGE ( 'NONE', *, *, #2459, .T. ) ;
#10391=VERTEX_POINT ( 'NONE', #13354 ) ;
#10392=LINE ( 'NONE', #8242, #5426 ) ;
#10395=CARTESIAN_POINT ( 'NONE',  ( -7.886584594865169606, -46.96511696614940234, 21.96004823855531640 ) ) ;
#10396=CARTESIAN_POINT ( 'NONE',  ( -7.796873843965146378, -46.67446211046079441, 47.00231026484400587 ) ) ;
#10405=ORIENTED_EDGE ( 'NONE', *, *, #5882, .T. ) ;
#10429=CARTESIAN_POINT ( 'NONE',  ( -20.69159174768329379, -22.05612254491840218, 56.64242933135466274 ) ) ;
#10431=LINE ( 'NONE', #13953, #6579 ) ;
#10438=ORIENTED_EDGE ( 'NONE', *, *, #4912, .T. ) ;
#10444=FACE_OUTER_BOUND ( 'NONE', #5525, .T. ) ;
#10452=( BOUNDED_CURVE ( )  B_SPLINE_CURVE ( 3, ( #2218, #8014, #7009, #8247 ),
 .UNSPECIFIED., .F., .T. ) 
 B_SPLINE_CURVE_WITH_KNOTS ( ( 4, 4 ),
 ( 1.628044839356179940, 3.141592653589792672 ),
 .UNSPECIFIED. ) 
 CURVE ( )  GEOMETRIC_REPRESENTATION_ITEM ( )  RATIONAL_B_SPLINE_CURVE ( ( 1.000000000000000000, 0.8180365063541270576, 0.8180365063541270576, 1.000000000000000000 ) ) 
 REPRESENTATION_ITEM ( '' )  );
#10460=CARTESIAN_POINT ( 'NONE',  ( -15.49969986081099904, -36.50737899243799944, -13.49768973515600479 ) ) ;
#10472=CARTESIAN_POINT ( 'NONE',  ( 2.500300139189001403, -46.50737899243799944, -2.497689735156001678 ) ) ;
#10474=DIRECTION ( 'NONE',  ( 1.000000000000000000, -1.291538348938060198E-32, 1.054621095516909827E-16 ) ) ;
#10483=ORIENTED_EDGE ( 'NONE', *, *, #11827, .F. ) ;
#10485=PRODUCT_DEFINITION_CONTEXT ( 'detailed design', #4297, 'design' ) ;
#10499=CARTESIAN_POINT ( 'NONE',  ( -23.08997828711216371, -47.08833727929018664, -17.22206101019868996 ) ) ;
#10502=CARTESIAN_POINT ( 'NONE',  ( 3.378223036541276425, -39.17044586890330038, -12.89965965032132011 ) ) ;
#10507=CARTESIAN_POINT ( 'NONE',  ( 3.575068303653157198, -38.90440891069084728, 51.78879027551830916 ) ) ;
#10514=CARTESIAN_POINT ( 'NONE',  ( -7.519596205739571104, -45.08052302622432705, 21.55821474351395750 ) ) ;
#10519=CARTESIAN_POINT ( 'NONE',  ( -15.49969986081099904, -27.00737899243800300, -13.49768973515600301 ) ) ;
#10525=CARTESIAN_POINT ( 'NONE',  ( -7.499699860810999041, -43.97742925780038092, -17.13441993860075385 ) ) ;
#10529=CARTESIAN_POINT ( 'NONE',  ( -12.85501980268021072, -23.15896895518548959, 56.90921755714956021 ) ) ;
#10533=CARTESIAN_POINT ( 'NONE',  ( -3.499699860810999041, -57.00737899243800655, 52.39987856403599409 ) ) ;
#10534=CYLINDRICAL_SURFACE ( 'NONE', #7494, 3.000000000000000000 ) ;
#10539=VERTEX_POINT ( 'NONE', #11075 ) ;
#10541=DIRECTION ( 'NONE',  ( 3.839882694219489529E-17, -1.000000000000000000, 0.000000000000000000 ) ) ;
#10542=FACE_BOUND ( 'NONE', #9309, .T. ) ;
#10557=EDGE_CURVE ( 'NONE', #13947, #7202, #7044, .T. ) ;
#10558=LINE ( 'NONE', #5880, #13291 ) ;
#10560=EDGE_LOOP ( 'NONE', ( #11560, #12462, #9178, #7779, #12485, #12559 ) ) ;
#10567=EDGE_CURVE ( 'NONE', #2754, #9043, #4112, .T. ) ;
#10569=EDGE_CURVE ( 'NONE', #14718, #5530, #5041, .T. ) ;
#10570=CARTESIAN_POINT ( 'NONE',  ( 0.5796456139481135361, -52.92803351767889097, -14.44614973369544586 ) ) ;
#10577=CARTESIAN_POINT ( 'NONE',  ( 2.884402102475247531, -40.07747304542361633, -13.18227376421650199 ) ) ;
#10581=CARTESIAN_POINT ( 'NONE',  ( 4.396918593460392266, -38.07367433586049543, 51.28992524861065050 ) ) ;
#10592=CARTESIAN_POINT ( 'NONE',  ( -7.664252951136423242, -48.41696643141921896, -7.111243861656096676 ) ) ;
#10593=CARTESIAN_POINT ( 'NONE',  ( -5.499699860811000818, -46.50737899243799944, 19.50231026484399877 ) ) ;
#10602=DIRECTION ( 'NONE',  ( 0.000000000000000000, 0.000000000000000000, -1.000000000000000000 ) ) ;
#10617=LINE ( 'NONE', #14291, #2428 ) ;
#10637=DIRECTION ( 'NONE',  ( 0.000000000000000000, -1.000000000000000000, -1.224646799147350002E-16 ) ) ;
#10639=VERTEX_POINT ( 'NONE', #13377 ) ;
#10642=ORIENTED_EDGE ( 'NONE', *, *, #14642, .F. ) ;
#10644=CARTESIAN_POINT ( 'NONE',  ( -15.49969986081099904, -32.00737899243799944, 19.50231026484400232 ) ) ;
#10648=EDGE_CURVE ( 'NONE', #818, #7911, #7768, .T. ) ;
#10650=CARTESIAN_POINT ( 'NONE',  ( 3.680269495751442577, -38.76197583039466110, -12.72242068341919286 ) ) ;
#10651=ADVANCED_FACE ( 'NONE', ( #13747 ), #3036, .F. ) ;
#10659=CARTESIAN_POINT ( 'NONE',  ( -18.51905911803493865, -23.07164644789430596, 56.88620726433236285 ) ) ;
#10670=CARTESIAN_POINT ( 'NONE',  ( -20.18599136182623965, -36.50737899243796392, 2.502310264844031629 ) ) ;
#10673=LINE ( 'NONE', #12984, #7121 ) ;
#10674=CARTESIAN_POINT ( 'NONE',  ( -16.02964405221278099, -52.50737899243799944, 57.00231026484399166 ) ) ;
#10680=PRODUCT_DEFINITION ( 'UNKNOWN', '', #6801, #10485 ) ;
#10687=CARTESIAN_POINT ( 'NONE',  ( 4.000300139189000959, -20.37340439622240851, 51.53354502093799994 ) ) ;
#10692=ORIENTED_EDGE ( 'NONE', *, *, #11672, .F. ) ;
#10695=DIRECTION ( 'NONE',  ( 1.000000000000000000, -1.291538348938060198E-32, 1.054621095516909827E-16 ) ) ;
#10697=AXIS2_PLACEMENT_3D ( 'NONE', #6100, #3976, #12011 ) ;
#10702=ADVANCED_FACE ( 'NONE', ( #5551 ), #3192, .F. ) ;
#10704=LINE ( 'NONE', #8403, #4302 ) ;
#10708=CARTESIAN_POINT ( 'NONE',  ( -33.88380182411292196, -40.07747304539473276, 52.18689429389564083 ) ) ;
#10715=ORIENTED_EDGE ( 'NONE', *, *, #8063, .T. ) ;
#10720=DIRECTION ( 'NONE',  ( 0.000000000000000000, 1.000000000000000000, 0.000000000000000000 ) ) ;
#10724=AXIS2_PLACEMENT_3D ( 'NONE', #8212, #2483, #4632 ) ;
#10725=CARTESIAN_POINT ( 'NONE',  ( -3.499699860810999041, -57.00737899243800655, -16.02584758213710003 ) ) ;
#10734=CARTESIAN_POINT ( 'NONE',  ( 3.273611621580635678, -39.31333522019950522, 51.96562901102289800 ) ) ;
#10745=CARTESIAN_POINT ( 'NONE',  ( -7.611722567307242393, -48.62974432432520189, -4.173814398520391045 ) ) ;
#10750=VERTEX_POINT ( 'NONE', #7618 ) ;
#10755=CARTESIAN_POINT ( 'NONE',  ( -18.80568317180454940, -37.21776555879632298, 56.85708068924256509 ) ) ;
#10758=CARTESIAN_POINT ( 'NONE',  ( -13.42625477939331624, -36.76308351228195193, -17.94383996831232864 ) ) ;
#10759=APPLICATION_CONTEXT ( 'automotive_design' ) ;
#10775=VERTEX_POINT ( 'NONE', #14817 ) ;
#10781=CARTESIAN_POINT ( 'NONE',  ( -33.49969986081099904, -42.00737899243800655, -13.39525803434800011 ) ) ;
#10799=VECTOR ( 'NONE', #8024, 1000.000000000000000 ) ;
#10803=CARTESIAN_POINT ( 'NONE',  ( -15.49969986081099194, -27.00737899243800300, 11.50231026484399877 ) ) ;
#10809=EDGE_LOOP ( 'NONE', ( #9601, #9634, #8203, #5110 ) ) ;
#10823=CARTESIAN_POINT ( 'NONE',  ( -7.629407442448592924, -48.55937836029033150, -4.069029971051592476 ) ) ;
#10824=ORIENTED_EDGE ( 'NONE', *, *, #1417, .T. ) ;
#10828=ORIENTED_EDGE ( 'NONE', *, *, #11305, .F. ) ;
#10837=CARTESIAN_POINT ( 'NONE',  ( -11.72862643632814716, -22.77130243382190500, 56.81215603131989411 ) ) ;
#10839=AXIS2_PLACEMENT_3D ( 'NONE', #5111, #9776, #12604 ) ;
#10841=DIRECTION ( 'NONE',  ( 0.000000000000000000, 0.000000000000000000, -1.000000000000000000 ) ) ;
#10844=CARTESIAN_POINT ( 'NONE',  ( -7.495514965259227225, -43.99345095228514424, -5.341653756843942169 ) ) ;
#10859=CARTESIAN_POINT ( 'NONE',  ( -7.526618194427099340, -48.92257192762229323, 18.84067492369451813 ) ) ;
#10863=CARTESIAN_POINT ( 'NONE',  ( -10.61529477037414715, -50.86499734049451149, -17.68083815942426895 ) ) ;
#10868=EDGE_CURVE ( 'NONE', #4941, #6874, #8359, .T. ) ;
#10875=DIRECTION ( 'NONE',  ( 1.000000000000000000, 0.000000000000000000, 0.000000000000000000 ) ) ;
#10893=DIRECTION ( 'NONE',  ( 1.054621095516909827E-16, 1.224646799147350002E-16, -1.000000000000000000 ) ) ;
#10909=CARTESIAN_POINT ( 'NONE',  ( -9.085271536259636349, -21.17909668945641499, 56.44940867462261025 ) ) ;
#10911=DIRECTION ( 'NONE',  ( 0.000000000000000000, 0.000000000000000000, -1.000000000000000000 ) ) ;
#10916=CARTESIAN_POINT ( 'NONE',  ( -7.512805849530849400, -44.04964101872670312, -5.955427708867301106 ) ) ;
#10926=ADVANCED_FACE ( 'NONE', ( #13715 ), #7805, .F. ) ;
#10932=ORIENTED_EDGE ( 'NONE', *, *, #9202, .T. ) ;
#10933=CARTESIAN_POINT ( 'NONE',  ( -11.49753086077415709, -51.43925603750204800, -17.78423269032954224 ) ) ;
#10954=AXIS2_PLACEMENT_3D ( 'NONE', #570, #14418, #6363 ) ;
#10957=FACE_BOUND ( 'NONE', #14311, .T. ) ;
#10972=ORIENTED_EDGE ( 'NONE', *, *, #6847, .T. ) ;
#10978=CARTESIAN_POINT ( 'NONE',  ( -21.34246172570263411, -49.97817515884320017, 56.54480789128852791 ) ) ;
#10982=EDGE_CURVE ( 'NONE', #10775, #4535, #5523, .T. ) ;
#10985=CARTESIAN_POINT ( 'NONE',  ( -11.91594154455664700, -22.84528331856323291, 56.83039675413429848 ) ) ;
#10988=DIRECTION ( 'NONE',  ( 0.000000000000000000, 0.000000000000000000, -1.000000000000000000 ) ) ;
#10989=ORIENTED_EDGE ( 'NONE', *, *, #13109, .T. ) ;
#11001=AXIS2_PLACEMENT_3D ( 'NONE', #5611, #2026, #6968 ) ;
#11004=VERTEX_POINT ( 'NONE', #6509 ) ;
#11011=ORIENTED_EDGE ( 'NONE', *, *, #5297, .F. ) ;
#11014=VERTEX_POINT ( 'NONE', #1221 ) ;
#11015=EDGE_CURVE ( 'NONE', #1385, #8470, #7010, .T. ) ;
#11017=CARTESIAN_POINT ( 'NONE',  ( -7.838622488183276893, -46.81654903479443419, -3.012281934724219123 ) ) ;
#11018=CARTESIAN_POINT ( 'NONE',  ( -15.49969986081099904, -26.50737899243800655, 57.00231026484399877 ) ) ;
#11025=LINE ( 'NONE', #2774, #6073 ) ;
#11050=CARTESIAN_POINT ( 'NONE',  ( -33.49969986081099904, -51.00737899243799944, 52.39987856403599409 ) ) ;
#11051=EDGE_CURVE ( 'NONE', #3278, #1260, #9028, .T. ) ;
#11064=CARTESIAN_POINT ( 'NONE',  ( -23.49969986081099904, -44.50737899243799944, 19.50231026484399877 ) ) ;
#11065=CYLINDRICAL_SURFACE ( 'NONE', #13292, 3.000000000000002665 ) ;
#11067=DIRECTION ( 'NONE',  ( -1.000000000000000000, -3.839882694219489529E-17, 0.000000000000000000 ) ) ;
#11075=CARTESIAN_POINT ( 'NONE',  ( 2.500300139188999182, -42.00737899243800655, -13.39525803434800011 ) ) ;
#11077=VECTOR ( 'NONE', #2814, 1000.000000000000000 ) ;
#11078=CARTESIAN_POINT ( 'NONE',  ( -7.499751500627867884, -49.00722532478560822, 19.47034365934475275 ) ) ;
#11085=ORIENTED_EDGE ( 'NONE', *, *, #12207, .T. ) ;
#11086=ORIENTED_EDGE ( 'NONE', *, *, #3733, .T. ) ;
#11087=CARTESIAN_POINT ( 'NONE',  ( -34.57446802530316887, -38.90440891063803974, -12.78416974581375065 ) ) ;
#11090=AXIS2_PLACEMENT_3D ( 'NONE', #7689, #1817, #13523 ) ;
#11101=DIRECTION ( 'NONE',  ( 0.000000000000000000, 1.224646799147350002E-16, -1.000000000000000000 ) ) ;
#11105=VERTEX_POINT ( 'NONE', #14488 ) ;
#11133=CARTESIAN_POINT ( 'NONE',  ( -14.45138012959125184, -36.57197769750143124, 56.98857378514258443 ) ) ;
#11137=CARTESIAN_POINT ( 'NONE',  ( -15.49969986081099904, -36.50737899243799944, 57.00231026484399877 ) ) ;
#11139=B_SPLINE_CURVE_WITH_KNOTS ( 'NONE', 3,
 ( #11260, #780, #5439, #8952 ),
 .UNSPECIFIED., .F., .F.,
 ( 4, 4 ),
 ( 0.8772132959648567541, 1.000000000000000000 ),
 .UNSPECIFIED. ) ;
#11141=CARTESIAN_POINT ( 'NONE',  ( -5.499699860811003482, -46.50737899243799944, 44.50231026484399877 ) ) ;
#11146=CARTESIAN_POINT ( 'NONE',  ( -5.499699860811003482, -46.50737899243799944, 44.50231026484399877 ) ) ;
#11156=VERTEX_POINT ( 'NONE', #795 ) ;
#11158=CARTESIAN_POINT ( 'NONE',  ( -7.586235653186040651, -45.66775839773830370, -3.133043233650827375 ) ) ;
#11159=CIRCLE ( 'NONE', #654, 37.50000000000000711 ) ;
#11164=CARTESIAN_POINT ( 'NONE',  ( -7.886584594865169606, -46.96511696614940234, 21.96004823855531640 ) ) ;
#11170=CARTESIAN_POINT ( 'NONE',  ( -8.710519834377311810, -48.73976024287854614, 45.63987292668604567 ) ) ;
#11171=PRODUCT ( 'Cross Slide Block', 'Cross Slide Block', '', ( #7770 ) ) ;
#11177=CARTESIAN_POINT ( 'NONE',  ( -7.515340099725619005, -44.00737978687738661, 44.36832752824940940 ) ) ;
#11183=CARTESIAN_POINT ( 'NONE',  ( -7.512159534862917099, -44.97983827236478049, -7.479109963946024564 ) ) ;
#11196=DIRECTION ( 'NONE',  ( -1.000000000000000000, 1.291538348938060198E-32, -1.054621095516909827E-16 ) ) ;
#11206=B_SPLINE_CURVE_WITH_KNOTS ( 'NONE', 3,
 ( #2135, #6930, #12544, #8080, #11614, #1130, #10238, #911, #9085, #5792 ),
 .UNSPECIFIED., .F., .F.,
 ( 4, 2, 2, 2, 4 ),
 ( 0.000000000000000000, 0.0005821621410504860704, 0.001164324282100972141, 0.001746486423151458103, 0.002328648564201944281 ),
 .UNSPECIFIED. ) ;
#11214=AXIS2_PLACEMENT_3D ( 'NONE', #3983, #14538, #14392 ) ;
#11215=FACE_OUTER_BOUND ( 'NONE', #2638, .T. ) ;
#11225=VERTEX_POINT ( 'NONE', #716 ) ;
#11233=CARTESIAN_POINT ( 'NONE',  ( -7.749729581312787552, -48.02091033735556636, 21.51272064359849168 ) ) ;
#11234=CARTESIAN_POINT ( 'NONE',  ( -15.49969986081099904, -52.50737899243800655, -13.49768973515600656 ) ) ;
#11244=CARTESIAN_POINT ( 'NONE',  ( -10.83521803515972159, -51.01205933293365291, 56.71172365652226688 ) ) ;
#11248=CARTESIAN_POINT ( 'NONE',  ( -8.309331736433431814, -48.01736933888442849, 46.50111227020314431 ) ) ;
#11252=ADVANCED_FACE ( 'NONE', ( #13716 ), #946, .F. ) ;
#11260=CARTESIAN_POINT ( 'NONE',  ( -7.754796638793765240, -46.50763592918296752, 17.00313569000094560 ) ) ;
#11265=CARTESIAN_POINT ( 'NONE',  ( -7.795459123704181259, -47.76474896896235123, -7.658500196163376295 ) ) ;
#11271=DIRECTION ( 'NONE',  ( 0.7071067811865475727, -0.7071067811865475727, -1.202263280131018653E-17 ) ) ;
#11273=ORIENTED_EDGE ( 'NONE', *, *, #11411, .F. ) ;
#11277=CARTESIAN_POINT ( 'NONE',  ( -10.21615383005687505, -38.47745445305465495, 56.63013494352767907 ) ) ;
#11283=CARTESIAN_POINT ( 'NONE',  ( -38.49969986081099904, -37.00737899243799944, 49.12071670408379731 ) ) ;
#11294=CARTESIAN_POINT ( 'NONE',  ( -18.07633053687676750, -36.92914190242253625, -17.90990850420651626 ) ) ;
#11299=DIRECTION ( 'NONE',  ( 1.445602896647337931E-16, 0.000000000000000000, -1.000000000000000000 ) ) ;
#11305=EDGE_CURVE ( 'NONE', #777, #9604, #1741, .T. ) ;
#11309=EDGE_CURVE ( 'NONE', #14890, #6515, #13982, .T. ) ;
#11310=CARTESIAN_POINT ( 'NONE',  ( -7.508831348196946642, -44.91519662196459706, -3.570265637683905702 ) ) ;
#11312=ORIENTED_EDGE ( 'NONE', *, *, #12608, .F. ) ;
#11315=CARTESIAN_POINT ( 'NONE',  ( -7.754798889200088752, -46.50763646577239285, -7.996864293225370623 ) ) ;
#11318=CIRCLE ( 'NONE', #2516, 37.50000000000000000 ) ;
#11330=ORIENTED_EDGE ( 'NONE', *, *, #11900, .F. ) ;
#11339=CARTESIAN_POINT ( 'NONE',  ( -23.49969986081099904, -44.50737899243799944, -109.5506571639849938 ) ) ;
#11346=CARTESIAN_POINT ( 'NONE',  ( -34.99969986081099904, -20.37340439622244048, -12.52892449124999885 ) ) ;
#11356=CARTESIAN_POINT ( 'NONE',  ( -7.499699860810998153, -44.50737899243799944, 56.13904046828873362 ) ) ;
#11360=CIRCLE ( 'NONE', #7200, 8.000000000000000000 ) ;
#11362=CYLINDRICAL_SURFACE ( 'NONE', #111, 2.500000000000000000 ) ;
#11363=DIRECTION ( 'NONE',  ( 0.000000000000000000, 0.000000000000000000, -1.000000000000000000 ) ) ;
#11366=CARTESIAN_POINT ( 'NONE',  ( -11.90127153857800657, -52.50737899243802786, 2.502310264844031185 ) ) ;
#11368=ORIENTED_EDGE ( 'NONE', *, *, #2386, .T. ) ;
#11370=DIRECTION ( 'NONE',  ( 0.000000000000000000, -1.000000000000000000, -1.224646799147350002E-16 ) ) ;
#11374=DIRECTION ( 'NONE',  ( 0.000000000000000000, 0.000000000000000000, 1.000000000000000000 ) ) ;
#11383=CARTESIAN_POINT ( 'NONE',  ( -7.503594565398491234, -44.64029237675795514, -3.819848327953776934 ) ) ;
#11385=CARTESIAN_POINT ( 'NONE',  ( -15.57469986081099478, -23.50737899243800300, 56.85231026484400019 ) ) ;
#11386=ORIENTED_EDGE ( 'NONE', *, *, #1417, .F. ) ;
#11392=LINE ( 'NONE', #7639, #10124 ) ;
#11411=EDGE_CURVE ( 'NONE', #9329, #6799, #8194, .T. ) ;
#11416=VECTOR ( 'NONE', #11934, 1000.000000000000000 ) ;
#11417=ORIENTED_EDGE ( 'NONE', *, *, #1537, .F. ) ;
#11419=CARTESIAN_POINT ( 'NONE',  ( -22.78941651591205186, -47.81319948894917360, -17.28247564077643261 ) ) ;
#11427=DIRECTION ( 'NONE',  ( 1.000000000000000000, -1.291538348938060198E-32, 1.054621095516909827E-16 ) ) ;
#11428=VERTEX_POINT ( 'NONE', #12881 ) ;
#11430=CARTESIAN_POINT ( 'NONE',  ( -7.909388035719858934, -41.92610292194794397, 56.22667989926442544 ) ) ;
#11444=DIRECTION ( 'NONE',  ( 0.000000000000000000, 0.000000000000000000, -1.000000000000000000 ) ) ;
#11450=AXIS2_PLACEMENT_3D ( 'NONE', #10593, #13054, #12899 ) ;
#11470=CYLINDRICAL_SURFACE ( 'NONE', #1033, 2.499999999999998668 ) ;
#11493=ADVANCED_FACE ( 'NONE', ( #548 ), #1845, .T. ) ;
#11494=ORIENTED_EDGE ( 'NONE', *, *, #10282, .F. ) ;
#11498=CARTESIAN_POINT ( 'NONE',  ( -5.499699860811000818, -46.50737899243799944, 19.50231026484399877 ) ) ;
#11499=ORIENTED_EDGE ( 'NONE', *, *, #9923, .F. ) ;
#11503=CARTESIAN_POINT ( 'NONE',  ( -7.512805849530849400, -44.04964101872660365, 19.96004823855532706 ) ) ;
#11506=DIRECTION ( 'NONE',  ( 0.000000000000000000, 1.850371707708594316E-16, -1.000000000000000000 ) ) ;
#11508=DIRECTION ( 'NONE',  ( -1.734723475976807094E-16, 0.000000000000000000, 1.000000000000000000 ) ) ;
#11516=ORIENTED_EDGE ( 'NONE', *, *, #5445, .F. ) ;
#11529=CARTESIAN_POINT ( 'NONE',  ( -5.499699860810998153, -46.50737899243799944, -5.497689735156003010 ) ) ;
#11531=AXIS2_PLACEMENT_3D ( 'NONE', #10041, #11427, #13652 ) ;
#11534=VECTOR ( 'NONE', #10541, 1000.000000000000000 ) ;
#11536=CARTESIAN_POINT ( 'NONE',  ( -15.49969986081099194, -27.00737899243800300, 19.50231026484399877 ) ) ;
#11550=DIRECTION ( 'NONE',  ( 0.000000000000000000, 0.000000000000000000, -1.000000000000000000 ) ) ;
#11559=ORIENTED_EDGE ( 'NONE', *, *, #11900, .T. ) ;
#11560=ORIENTED_EDGE ( 'NONE', *, *, #7482, .F. ) ;
#11564=ORIENTED_EDGE ( 'NONE', *, *, #12788, .F. ) ;
#11566=ADVANCED_FACE ( 'NONE', ( #7500, #10957, #1922 ), #14547, .T. ) ;
#11567=DIRECTION ( 'NONE',  ( 1.000000000000000000, -1.291538348938060198E-32, 1.054621095516909827E-16 ) ) ;
#11569=EDGE_CURVE ( 'NONE', #13213, #6631, #12705, .T. ) ;
#11570=CARTESIAN_POINT ( 'NONE',  ( -22.29355530218780501, -48.73954551910809840, -17.37742864379163876 ) ) ;
#11577=CARTESIAN_POINT ( 'NONE',  ( 2.510125670910141160, -41.64595657060088740, 52.39450821273811698 ) ) ;
#11579=CARTESIAN_POINT ( 'NONE',  ( -20.85440823583763859, -21.95508377545333900, 56.61960193865294144 ) ) ;
#11581=DIRECTION ( 'NONE',  ( 0.000000000000000000, -1.000000000000000000, -1.224646799147350002E-16 ) ) ;
#11584=AXIS2_PLACEMENT_3D ( 'NONE', #12975, #5013, #13205 ) ;
#11591=CARTESIAN_POINT ( 'NONE',  ( -7.568963286690253867, -45.57243725087103314, 42.17552517324416783 ) ) ;
#11601=AXIS2_PLACEMENT_3D ( 'NONE', #14947, #1102, #6899 ) ;
#11614=CARTESIAN_POINT ( 'NONE',  ( -7.568637282891814699, -45.56971093230124836, 46.82783525944628877 ) ) ;
#11616=CARTESIAN_POINT ( 'NONE',  ( -7.495514965259227225, -43.99345095228513713, 19.34627428653194769 ) ) ;
#11618=LINE ( 'NONE', #12783, #14228 ) ;
#11621=CARTESIAN_POINT ( 'NONE',  ( -38.20335605883195029, -37.00737899243799234, 49.35084074737085302 ) ) ;
#11622=DIRECTION ( 'NONE',  ( -0.4999999999999998890, 0.8660254037844387076, 0.000000000000000000 ) ) ;
#11631=ADVANCED_FACE ( 'NONE', ( #10251 ), #4289, .T. ) ;
#11637=CYLINDRICAL_SURFACE ( 'NONE', #5625, 8.000000000000000000 ) ;
#11647=VERTEX_POINT ( 'NONE', #1000 ) ;
#11651=CARTESIAN_POINT ( 'NONE',  ( 6.329928126373893349, -37.10979894228395182, 50.00103417101053083 ) ) ;
#11656=CARTESIAN_POINT ( 'NONE',  ( -23.49969986081099904, -44.50737899243799944, 19.50231026484399877 ) ) ;
#11658=CARTESIAN_POINT ( 'NONE',  ( -33.49969986081099904, -51.00737899243799944, 19.50231026484398456 ) ) ;
#11660=LINE ( 'NONE', #5018, #13160 ) ;
#11671=VERTEX_POINT ( 'NONE', #3141 ) ;
#11672=EDGE_CURVE ( 'NONE', #3526, #10020, #8620, .T. ) ;
#11675=CARTESIAN_POINT ( 'NONE',  ( -14.71582029074517095, -23.50178099748875837, 57.00081750421114890 ) ) ;
#11696=DIRECTION ( 'NONE',  ( 0.000000000000000000, 0.000000000000000000, 1.000000000000000000 ) ) ;
#11698=CARTESIAN_POINT ( 'NONE',  ( -35.37586185869766808, -38.10176464241880012, 51.30163939567694342 ) ) ;
#11702=UNCERTAINTY_MEASURE_WITH_UNIT (LENGTH_MEASURE( 1.000000000000000082E-05 ), #10339, 'distance_accuracy_value', 'NONE');
#11706=CARTESIAN_POINT ( 'NONE',  ( -15.49969986081099904, -57.00737899243800655, 19.50231026484399877 ) ) ;
#11711=ORIENTED_EDGE ( 'NONE', *, *, #6343, .F. ) ;
#11725=CARTESIAN_POINT ( 'NONE',  ( 3.682457005310663334, -38.77348753606410270, 51.72516835908339772 ) ) ;
#11736=DIRECTION ( 'NONE',  ( 0.000000000000000000, -1.000000000000000000, -1.224646799147350002E-16 ) ) ;
#11738=ORIENTED_EDGE ( 'NONE', *, *, #5233, .F. ) ;
#11744=PRESENTATION_STYLE_ASSIGNMENT (( #7144 ) ) ;
#11745=ORIENTED_EDGE ( 'NONE', *, *, #9923, .T. ) ;
#11752=ORIENTED_EDGE ( 'NONE', *, *, #2059, .T. ) ;
#11765=CARTESIAN_POINT ( 'NONE',  ( -7.949896068685645467, -47.15850730160504867, 46.92147361607200651 ) ) ;
#11775=CARTESIAN_POINT ( 'NONE',  ( -23.49969986081099904, -19.50737899243800300, 48.00231026484399877 ) ) ;
#11784=ORIENTED_EDGE ( 'NONE', *, *, #4879, .T. ) ;
#11785=AXIS2_PLACEMENT_3D ( 'NONE', #6913, #12677, #11444 ) ;
#11799=CARTESIAN_POINT ( 'NONE',  ( 4.595282735339393909, -37.93213861349479288, -12.15966626606534717 ) ) ;
#11800=ORIENTED_EDGE ( 'NONE', *, *, #4912, .F. ) ;
#11803=VERTEX_POINT ( 'NONE', #13169 ) ;
#11812=VECTOR ( 'NONE', #4410, 1000.000000000000000 ) ;
#11814=CARTESIAN_POINT ( 'NONE',  ( -7.504576870302558156, -44.41851609332119466, 20.88336806361667897 ) ) ;
#11815=CYLINDRICAL_SURFACE ( 'NONE', #11450, 2.999999999999999112 ) ;
#11820=EDGE_LOOP ( 'NONE', ( #14194, #9662 ) ) ;
#11824=ORIENTED_EDGE ( 'NONE', *, *, #5335, .F. ) ;
#11827=EDGE_CURVE ( 'NONE', #5287, #5522, #1876, .T. ) ;
#11837=CARTESIAN_POINT ( 'NONE',  ( -15.49969986081099904, -13.50737899243800122, 54.00231026484400587 ) ) ;
#11847=LINE ( 'NONE', #153, #4041 ) ;
#11854=FACE_OUTER_BOUND ( 'NONE', #648, .T. ) ;
#11855=CARTESIAN_POINT ( 'NONE',  ( -37.02289807341878713, -37.22897031456928119, 50.21085258507981308 ) ) ;
#11860=DIRECTION ( 'NONE',  ( 0.000000000000000000, 1.850371707708594316E-16, -1.000000000000000000 ) ) ;
#11868=DIRECTION ( 'NONE',  ( 0.000000000000000000, -1.000000000000000000, -1.224646799147350002E-16 ) ) ;
#11874=CARTESIAN_POINT ( 'NONE',  ( 2.500300139189003623, -41.64411882298843892, -13.39525803434795570 ) ) ;
#11890=CARTESIAN_POINT ( 'NONE',  ( -7.649802761028805520, -48.47628348355120664, -3.956830880212969248 ) ) ;
#11898=DIRECTION ( 'NONE',  ( 1.000000000000000000, -1.291538348938060198E-32, 1.054621095516909827E-16 ) ) ;
#11900=EDGE_CURVE ( 'NONE', #5530, #3694, #3183, .T. ) ;
#11902=CARTESIAN_POINT ( 'NONE',  ( -10.83829729829802169, -38.00046876589347278, -17.70749226439889412 ) ) ;
#11903=B_SPLINE_CURVE_WITH_KNOTS ( 'NONE', 3,
 ( #12754, #7915, #4487, #10370, #14892, #8991, #11294, #4415, #823, #1113, #5626, #3336, #9067, #10293, #13743, #5703, #13673, #7987, #14964, #5772, #15037, #3486, #4561 ),
 .UNSPECIFIED., .F., .F.,
 ( 4, 2, 1, 2, 2, 2, 2, 2, 2, 2, 2, 4 ),
 ( 0.01260730609128223219, 0.01339570877218145863, 0.01418411145308068333, 0.01497251413397990977, 0.01576091681487913621, 0.01733772217667757867, 0.01891452753847602461, 0.02049133290027446708, 0.02127973558117368311, 0.02206813826207289914, 0.02364494362387132426, 0.02522174898566975285 ),
 .UNSPECIFIED. ) ;
#11904=VECTOR ( 'NONE', #2306, 1000.000000000000000 ) ;
#11916=CARTESIAN_POINT ( 'NONE',  ( -7.510805280342158774, -44.08454818175437850, 18.85714484343347408 ) ) ;
#11922=CYLINDRICAL_SURFACE ( 'NONE', #790, 8.000000000000000000 ) ;
#11923=DIRECTION ( 'NONE',  ( 0.000000000000000000, -1.000000000000000000, -1.224646799147350002E-16 ) ) ;
#11925=AXIS2_PLACEMENT_3D ( 'NONE', #13738, #8984, #10288 ) ;
#11934=DIRECTION ( 'NONE',  ( 0.000000000000000000, 0.000000000000000000, -1.000000000000000000 ) ) ;
#11935=CARTESIAN_POINT ( 'NONE',  ( -33.49969986081099904, -42.00737899243800655, 52.39987856403599409 ) ) ;
#11937=AXIS2_PLACEMENT_3D ( 'NONE', #12747, #8910, #4254 ) ;
#11938=ORIENTED_EDGE ( 'NONE', *, *, #10569, .T. ) ;
#11939=CARTESIAN_POINT ( 'NONE',  ( -7.501944906337848273, -44.50613385756380325, -4.001965388595783324 ) ) ;
#11940=VERTEX_POINT ( 'NONE', #2995 ) ;
#11957=CARTESIAN_POINT ( 'NONE',  ( 4.194495296137883855, -38.25609885807656951, -12.40989724287477891 ) ) ;
#11962=CARTESIAN_POINT ( 'NONE',  ( 3.853695978508554720, -38.58518656693815529, 51.62240523568905104 ) ) ;
#11981=FACE_OUTER_BOUND ( 'NONE', #8543, .T. ) ;
#11982=ORIENTED_EDGE ( 'NONE', *, *, #177, .T. ) ;
#11983=FACE_OUTER_BOUND ( 'NONE', #10560, .T. ) ;
#11987=CARTESIAN_POINT ( 'NONE',  ( -9.097666755470994460, -21.18944696257707250, 56.45155857467202054 ) ) ;
#11988=UNCERTAINTY_MEASURE_WITH_UNIT (LENGTH_MEASURE( 1.000000000000000082E-05 ), #14278, 'distance_accuracy_value', 'NONE');
#12007=CARTESIAN_POINT ( 'NONE',  ( -7.804240102366953202, -47.71020347972454090, 17.31052141267318234 ) ) ;
#12010=CARTESIAN_POINT ( 'NONE',  ( -15.49969986081099371, -52.50737899243799944, -17.99768973515599768 ) ) ;
#12011=DIRECTION ( 'NONE',  ( 0.000000000000000000, 0.000000000000000000, -1.000000000000000000 ) ) ;
#12016=ORIENTED_EDGE ( 'NONE', *, *, #3083, .F. ) ;
#12019=ORIENTED_EDGE ( 'NONE', *, *, #8796, .T. ) ;
#12022=EDGE_CURVE ( 'NONE', #7911, #6717, #11318, .T. ) ;
#12024=( BOUNDED_CURVE ( )  B_SPLINE_CURVE ( 3, ( #14684, #6784, #7936, #8787 ),
 .UNSPECIFIED., .F., .T. ) 
 B_SPLINE_CURVE_WITH_KNOTS ( ( 4, 4 ),
 ( 2.168404344971017989E-16, 1.513547814233613842 ),
 .UNSPECIFIED. ) 
 CURVE ( )  GEOMETRIC_REPRESENTATION_ITEM ( )  RATIONAL_B_SPLINE_CURVE ( ( 1.000000000000000000, 0.8180365063541268356, 0.8180365063541268356, 1.000000000000000000 ) ) 
 REPRESENTATION_ITEM ( '' )  );
#12035=ORIENTED_EDGE ( 'NONE', *, *, #3908, .F. ) ;
#12053=CARTESIAN_POINT ( 'NONE',  ( -15.49969986081099194, -52.50737899243800655, 11.50231026484399521 ) ) ;
#12056=ORIENTED_EDGE ( 'NONE', *, *, #3966, .F. ) ;
#12068=AXIS2_PLACEMENT_3D ( 'NONE', #11385, #1982, #12621 ) ;
#12073=CYLINDRICAL_SURFACE ( 'NONE', #2859, 10.00000000000000000 ) ;
#12077=EDGE_LOOP ( 'NONE', ( #7579, #7459, #5813, #5459 ) ) ;
#12078=CARTESIAN_POINT ( 'NONE',  ( -15.57469986081567370, -23.50709773848280904, 57.00223526477360281 ) ) ;
#12083=CARTESIAN_POINT ( 'NONE',  ( -7.499960972858382924, -49.00661531336379539, 19.43850304437339460 ) ) ;
#12087=EDGE_LOOP ( 'NONE', ( #5980, #6813, #14064, #11494 ) ) ;
#12089=CARTESIAN_POINT ( 'NONE',  ( -33.53940702758666248, -41.28381732916982827, 52.37824589759239302 ) ) ;
#12091=ORIENTED_EDGE ( 'NONE', *, *, #3908, .T. ) ;
#12092=CARTESIAN_POINT ( 'NONE',  ( -7.512805849530849400, -44.04964101872660365, -5.039951761444699585 ) ) ;
#12094=CARTESIAN_POINT ( 'NONE',  ( -36.64373166576667273, -37.36437517128344155, -11.46837648659897546 ) ) ;
#12102=DIRECTION ( 'NONE',  ( 0.000000000000000000, 0.000000000000000000, -1.000000000000000000 ) ) ;
#12103=EDGE_CURVE ( 'NONE', #7229, #13194, #2769, .T. ) ;
#12112=VERTEX_POINT ( 'NONE', #5055 ) ;
#12115=CARTESIAN_POINT ( 'NONE',  ( 2.500300139188999182, -51.00737899243799944, -13.39525803434800011 ) ) ;
#12132=CARTESIAN_POINT ( 'NONE',  ( -11.30912773046065922, -22.58799119088164886, 56.76750275176264182 ) ) ;
#12146=CIRCLE ( 'NONE', #5537, 2.999999999999999112 ) ;
#12147=AXIS2_PLACEMENT_3D ( 'NONE', #3803, #1658, #1358 ) ;
#12150=CARTESIAN_POINT ( 'NONE',  ( -7.671650320578238258, -48.38766871647332835, 17.85456079179654765 ) ) ;
#12152=EDGE_CURVE ( 'NONE', #2093, #3246, #10558, .T. ) ;
#12157=CARTESIAN_POINT ( 'NONE',  ( -33.99488797801397055, -39.83604612059843930, 52.12407946957260663 ) ) ;
#12162=VECTOR ( 'NONE', #14937, 1000.000000000000000 ) ;
#12163=CARTESIAN_POINT ( 'NONE',  ( -33.88323046362949498, -40.08477038825456873, -13.18250565558182785 ) ) ;
#12164=ORIENTED_EDGE ( 'NONE', *, *, #515, .F. ) ;
#12175=EDGE_CURVE ( 'NONE', #8446, #11671, #2266, .T. ) ;
#12176=CARTESIAN_POINT ( 'NONE',  ( -15.49969986081099194, -57.00737899243800655, 19.50231026484398811 ) ) ;
#12186=ORIENTED_EDGE ( 'NONE', *, *, #16, .T. ) ;
#12201=EDGE_LOOP ( 'NONE', ( #4908, #5290, #798, #10405, #755, #9697 ) ) ;
#12205=AXIS2_PLACEMENT_3D ( 'NONE', #13066, #6076, #7304 ) ;
#12207=EDGE_CURVE ( 'NONE', #1735, #11004, #4051, .T. ) ;
#12214=VERTEX_POINT ( 'NONE', #5126 ) ;
#12223=CARTESIAN_POINT ( 'NONE',  ( -31.57904533557010751, -52.92803351767889097, 53.45077026338344695 ) ) ;
#12227=ADVANCED_FACE ( 'NONE', ( #681 ), #13324, .F. ) ;
#12231=AXIS2_PLACEMENT_3D ( 'NONE', #12417, #11567, #10182 ) ;
#12237=ORIENTED_EDGE ( 'NONE', *, *, #3956, .F. ) ;
#12239=CARTESIAN_POINT ( 'NONE',  ( -36.69937278055155616, -37.34275670915150869, -11.43026766154685703 ) ) ;
#12241=VERTEX_POINT ( 'NONE', #5417 ) ;
#12252=LINE ( 'NONE', #6565, #9683 ) ;
#12256=ORIENTED_EDGE ( 'NONE', *, *, #9844, .F. ) ;
#12266=EDGE_CURVE ( 'NONE', #6717, #9043, #12806, .T. ) ;
#12284=DIRECTION ( 'NONE',  ( 1.000000000000000000, 0.000000000000000000, 0.000000000000000000 ) ) ;
#12296=ADVANCED_FACE ( 'NONE', ( #4581 ), #2211, .F. ) ;
#12300=ORIENTED_EDGE ( 'NONE', *, *, #4513, .T. ) ;
#12314=ORIENTED_EDGE ( 'NONE', *, *, #2278, .T. ) ;
#12326=CARTESIAN_POINT ( 'NONE',  ( -5.499699860811000818, -46.50737899243799944, 19.50231026484399877 ) ) ;
#12329=CARTESIAN_POINT ( 'NONE',  ( -27.49969986081100259, -57.00737899243800655, 19.50231026484398811 ) ) ;
#12335=EDGE_CURVE ( 'NONE', #11004, #13213, #11206, .T. ) ;
#12337=CYLINDRICAL_SURFACE ( 'NONE', #13067, 8.000000000000000000 ) ;
#12342=CARTESIAN_POINT ( 'NONE',  ( -15.49969986081098838, -17.75737899243799944, 54.00231026484400587 ) ) ;
#12344=CARTESIAN_POINT ( 'NONE',  ( -7.804240102366930998, -47.71020347972489617, -7.689478587326622261 ) ) ;
#12355=CARTESIAN_POINT ( 'NONE',  ( -22.00675222451046409, -49.16858233193156735, 56.43373460882509818 ) ) ;
#12356=VERTEX_POINT ( 'NONE', #5862 ) ;
#12371=PLANE ( 'NONE',  #1523 ) ;
#12382=ORIENTED_EDGE ( 'NONE', *, *, #8697, .F. ) ;
#12383=DIRECTION ( 'NONE',  ( -1.000000000000000000, 1.291538348938060198E-32, -1.054621095516909827E-16 ) ) ;
#12384=CARTESIAN_POINT ( 'NONE',  ( -7.640804079088249878, -45.98079939124116322, -3.051398076617611643 ) ) ;
#12388=ORIENTED_EDGE ( 'NONE', *, *, #5588, .F. ) ;
#12392=CARTESIAN_POINT ( 'NONE',  ( -7.769540243250969702, -46.58425354491494375, 56.19700617964608114 ) ) ;
#12405=EDGE_LOOP ( 'NONE', ( #9194, #11711, #1026, #7912 ) ) ;
#12410=CARTESIAN_POINT ( 'NONE',  ( -34.99969986081099904, -20.37340439622244048, 51.53354502093799994 ) ) ;
#12413=DIRECTION ( 'NONE',  ( 0.000000000000000000, -1.000000000000000000, -1.224646799147350002E-16 ) ) ;
#12417=CARTESIAN_POINT ( 'NONE',  ( -5.499699860810998153, -46.50737899243799944, -5.497689735156003010 ) ) ;
#12418=AXIS2_PLACEMENT_3D ( 'NONE', #5207, #12102, #7573 ) ;
#12419=DIRECTION ( 'NONE',  ( 0.000000000000000000, 0.000000000000000000, 1.000000000000000000 ) ) ;
#12428=ORIENTED_EDGE ( 'NONE', *, *, #13750, .T. ) ;
#12432=EDGE_CURVE ( 'NONE', #7870, #5530, #6828, .T. ) ;
#12439=DIRECTION ( 'NONE',  ( -1.000000000000000000, 1.291538348938060198E-32, -1.054621095516909827E-16 ) ) ;
#12462=ORIENTED_EDGE ( 'NONE', *, *, #3733, .F. ) ;
#12463=LINE ( 'NONE', #4048, #4585 ) ;
#12464=CARTESIAN_POINT ( 'NONE',  ( -23.49969986081102036, -49.19367049345326848, -10.18398123617125428 ) ) ;
#12480=VERTEX_POINT ( 'NONE', #1442 ) ;
#12484=CARTESIAN_POINT ( 'NONE',  ( -7.541197117963764462, -45.30952225410057110, -7.694240868337988815 ) ) ;
#12485=ORIENTED_EDGE ( 'NONE', *, *, #11411, .T. ) ;
#12490=FACE_OUTER_BOUND ( 'NONE', #12077, .T. ) ;
#12493=CARTESIAN_POINT ( 'NONE',  ( -30.62513859619093637, -27.95036676736707548, -14.90232471354688037 ) ) ;
#12494=ORIENTED_EDGE ( 'NONE', *, *, #13441, .F. ) ;
#12497=DIRECTION ( 'NONE',  ( 0.000000000000000000, 1.700257036304450134E-17, -1.000000000000000000 ) ) ;
#12499=ORIENTED_EDGE ( 'NONE', *, *, #8697, .T. ) ;
#12509=CARTESIAN_POINT ( 'NONE',  ( -20.18599136182623965, -36.50737899243796392, 27.50231026484402719 ) ) ;
#12516=ORIENTED_EDGE ( 'NONE', *, *, #13986, .T. ) ;
#12531=CARTESIAN_POINT ( 'NONE',  ( -7.886584594865169606, -46.96511696614940234, 21.96004823855531640 ) ) ;
#12535=DIRECTION ( 'NONE',  ( 3.839882694219489529E-17, -1.000000000000000000, 0.000000000000000000 ) ) ;
#12539=CARTESIAN_POINT ( 'NONE',  ( -7.527660810972179206, -45.17397571328393013, -3.380064858389232985 ) ) ;
#12542=EDGE_CURVE ( 'NONE', #4535, #6874, #5701, .T. ) ;
#12544=CARTESIAN_POINT ( 'NONE',  ( -7.663319311905077313, -46.12821245145848792, 46.98080104517658384 ) ) ;
#12546=ORIENTED_EDGE ( 'NONE', *, *, #5133, .T. ) ;
#12548=CARTESIAN_POINT ( 'NONE',  ( 1.872105016583406778, -24.05954647699557114, -13.82452877272129399 ) ) ;
#12549=CARTESIAN_POINT ( 'NONE',  ( -7.550611734114103690, -45.55128411564821533, 56.15027137728581863 ) ) ;
#12554=CARTESIAN_POINT ( 'NONE',  ( -8.185397854257590922, -47.75120526332403159, 42.32787638714851397 ) ) ;
#12559=ORIENTED_EDGE ( 'NONE', *, *, #8424, .T. ) ;
#12563=CARTESIAN_POINT ( 'NONE',  ( -7.499699860810999041, -44.50737899243799944, -109.5506571639849938 ) ) ;
#12567=EDGE_CURVE ( 'NONE', #9329, #2702, #4517, .T. ) ;
#12568=CARTESIAN_POINT ( 'NONE',  ( -32.87150473820536689, -24.05954647699559601, 52.82914930240931994 ) ) ;
#12571=CARTESIAN_POINT ( 'NONE',  ( -15.49969986081099904, -27.00737899243800300, -13.49768973515600301 ) ) ;
#12572=AXIS2_PLACEMENT_3D ( 'NONE', #1161, #461, #8702 ) ;
#12573=CYLINDRICAL_SURFACE ( 'NONE', #12231, 3.000000000000000000 ) ;
#12574=EDGE_CURVE ( 'NONE', #12480, #9659, #14519, .T. ) ;
#12575=ORIENTED_EDGE ( 'NONE', *, *, #13109, .F. ) ;
#12582=DIRECTION ( 'NONE',  ( 0.000000000000000000, 0.000000000000000000, -1.000000000000000000 ) ) ;
#12587=VERTEX_POINT ( 'NONE', #1892 ) ;
#12604=DIRECTION ( 'NONE',  ( 0.000000000000000000, 0.000000000000000000, -1.000000000000000000 ) ) ;
#12605=ORIENTED_EDGE ( 'NONE', *, *, #2495, .T. ) ;
#12608=EDGE_CURVE ( 'NONE', #5496, #4806, #8700, .T. ) ;
#12621=DIRECTION ( 'NONE',  ( -3.839882694219489529E-17, 1.000000000000000000, 0.000000000000000000 ) ) ;
#12622=ORIENTED_EDGE ( 'NONE', *, *, #5335, .T. ) ;
#12623=CARTESIAN_POINT ( 'NONE',  ( -2.716578225681299141, -32.00737899243799944, -15.75165123257469801 ) ) ;
#12624=CARTESIAN_POINT ( 'NONE',  ( -10.62325334976782720, -50.85476156143290183, 56.68445949013308649 ) ) ;
#12627=CARTESIAN_POINT ( 'NONE',  ( -8.005579240875389857, -47.31158775777677761, 42.12977053007920603 ) ) ;
#12630=EDGE_CURVE ( 'NONE', #8099, #12721, #4002, .T. ) ;
#12646=CARTESIAN_POINT ( 'NONE',  ( 4.000300139189000959, -20.37340439622242982, -17.99768973515599768 ) ) ;
#12648=DIRECTION ( 'NONE',  ( 1.054621095516909827E-16, 1.224646799147350002E-16, -1.000000000000000000 ) ) ;
#12665=AXIS2_PLACEMENT_3D ( 'NONE', #226, #9400, #3890 ) ;
#12667=CARTESIAN_POINT ( 'NONE',  ( -15.49969986081099194, -36.50737899243799944, 11.50231026484399699 ) ) ;
#12677=DIRECTION ( 'NONE',  ( 0.000000000000000000, -1.000000000000000000, -1.224646799147350002E-16 ) ) ;
#12681=EDGE_CURVE ( 'NONE', #12888, #2185, #7916, .T. ) ;
#12696=ORIENTED_EDGE ( 'NONE', *, *, #14406, .T. ) ;
#12705=B_SPLINE_CURVE_WITH_KNOTS ( 'NONE', 3,
 ( #13406, #5284, #5137, #6275, #483, #9801, #6568, #1693, #7575, #11177, #3990, #13554, #3915, #14619, #2918, #623, #3059, #697 ),
 .UNSPECIFIED., .F., .F.,
 ( 4, 2, 2, 2, 2, 2, 2, 2, 4 ),
 ( 0.002328648564201944281, 0.002729030124645695152, 0.003129411685089445588, 0.003529793245533196459, 0.003930174805976947329, 0.004330556366420697766, 0.004730937926864449070, 0.005131319487308199506, 0.005531701047751949943 ),
 .UNSPECIFIED. ) ;
#12721=VERTEX_POINT ( 'NONE', #10294 ) ;
#12722=DIRECTION ( 'NONE',  ( -1.000000000000000000, 0.000000000000000000, 0.000000000000000000 ) ) ;
#12732=ORIENTED_EDGE ( 'NONE', *, *, #4124, .F. ) ;
#12733=DIRECTION ( 'NONE',  ( 1.000000000000000000, -1.291538348938060198E-32, 1.054621095516909827E-16 ) ) ;
#12747=CARTESIAN_POINT ( 'NONE',  ( 2.500300139188999182, -37.00737899243799944, 19.50231026484398811 ) ) ;
#12749=CARTESIAN_POINT ( 'NONE',  ( -7.517356049973301424, -45.05918421631233173, 42.45528228030804030 ) ) ;
#12754=CARTESIAN_POINT ( 'NONE',  ( -15.49969986081099371, -36.50737899243799944, -17.99768973515599768 ) ) ;
#12756=ORIENTED_EDGE ( 'NONE', *, *, #684, .T. ) ;
#12764=MANIFOLD_SOLID_BREP ( 'Stock-MAS-672-1', #8519 ) ;
#12776=AXIS2_PLACEMENT_3D ( 'NONE', #4134, #919, #10319 ) ;
#12779=DIRECTION ( 'NONE',  ( 0.000000000000000000, -9.251858538542971581E-17, 1.000000000000000000 ) ) ;
#12783=CARTESIAN_POINT ( 'NONE',  ( -5.499699860811000818, -46.50737899243799944, 16.50231026484399877 ) ) ;
#12788=EDGE_CURVE ( 'NONE', #14718, #12356, #6248, .T. ) ;
#12799=ORIENTED_EDGE ( 'NONE', *, *, #2707, .F. ) ;
#12802=CIRCLE ( 'NONE', #1548, 2.999999999999999112 ) ;
#12806=CIRCLE ( 'NONE', #104, 37.50000000000000000 ) ;
#12811=CARTESIAN_POINT ( 'NONE',  ( 4.791762596210716652, -37.80121036461403605, -12.03389752085011644 ) ) ;
#12812=EDGE_LOOP ( 'NONE', ( #3229, #8637, #9216, #12816, #8857, #9337, #11745, #13175 ) ) ;
#12815=EDGE_LOOP ( 'NONE', ( #6479, #1872, #1185, #7060, #13576, #4529, #8911, #11559 ) ) ;
#12816=ORIENTED_EDGE ( 'NONE', *, *, #7474, .F. ) ;
#12817=CARTESIAN_POINT ( 'NONE',  ( 4.049098414795642142, -38.38910658709895074, 51.50382295336648752 ) ) ;
#12819=CARTESIAN_POINT ( 'NONE',  ( -20.16941728185991423, -22.35032937287301991, 56.71056454896548615 ) ) ;
#12830=DIRECTION ( 'NONE',  ( -1.000000000000000000, 1.291538348938060198E-32, -1.054621095516909827E-16 ) ) ;
#12831=DIRECTION ( 'NONE',  ( 0.000000000000000000, -1.000000000000000000, -1.224646799147350002E-16 ) ) ;
#12835=CARTESIAN_POINT ( 'NONE',  ( -22.43956949979004634, -40.49372917221637636, 56.35573215670456193 ) ) ;
#12837=( BOUNDED_CURVE ( )  B_SPLINE_CURVE ( 3, ( #23, #10570, #3533, #10725 ),
 .UNSPECIFIED., .F., .F. ) 
 B_SPLINE_CURVE_WITH_KNOTS ( ( 4, 4 ),
 ( 1.070141614390309526, 1.245066839500267530 ),
 .UNSPECIFIED. ) 
 CURVE ( )  GEOMETRIC_REPRESENTATION_ITEM ( )  RATIONAL_B_SPLINE_CURVE ( ( 1.000000000000000000, 0.9974517222217440526, 0.9974517222217440526, 1.000000000000000000 ) ) 
 REPRESENTATION_ITEM ( '' )  );
#12838=CARTESIAN_POINT ( 'NONE',  ( -10.62581258585845667, -38.15807761791479180, -17.68017016644601114 ) ) ;
#12843=ADVANCED_FACE ( 'NONE', ( #11983 ), #12337, .F. ) ;
#12844=LINE ( 'NONE', #6992, #9670 ) ;
#12850=CARTESIAN_POINT ( 'NONE',  ( -23.49969986081100259, -44.50737899243799944, -17.13441993860073254 ) ) ;
#12852=ORIENTED_EDGE ( 'NONE', *, *, #12335, .T. ) ;
#12861=CARTESIAN_POINT ( 'NONE',  ( -7.719139325354606562, -48.17958124988514612, -7.357509729390519837 ) ) ;
#12862=CARTESIAN_POINT ( 'NONE',  ( -36.48074150599295962, -37.42264482913270740, 50.58571613516381404 ) ) ;
#12879=AXIS2_PLACEMENT_3D ( 'NONE', #3815, #9630, #9781 ) ;
#12881=CARTESIAN_POINT ( 'NONE',  ( -23.49969986081099904, -19.50737899243800300, 54.00231026484400587 ) ) ;
#12886=ORIENTED_EDGE ( 'NONE', *, *, #4857, .F. ) ;
#12887=CARTESIAN_POINT ( 'NONE',  ( 5.757201503570998469, -37.32104008884124369, 50.39558766532553591 ) ) ;
#12888=VERTEX_POINT ( 'NONE', #8953 ) ;
#12898=CARTESIAN_POINT ( 'NONE',  ( 2.500300139189001847, -46.50737899243799944, -5.497689735156002122 ) ) ;
#12899=DIRECTION ( 'NONE',  ( 0.000000000000000000, 0.000000000000000000, -1.000000000000000000 ) ) ;
#12905=ORIENTED_EDGE ( 'NONE', *, *, #11569, .F. ) ;
#12928=VERTEX_POINT ( 'NONE', #2823 ) ;
#12936=DIRECTION ( 'NONE',  ( 0.000000000000000000, -1.000000000000000000, -1.224646799147350002E-16 ) ) ;
#12939=CARTESIAN_POINT ( 'NONE',  ( -23.49969986081099904, -19.50737899243800300, 54.00231026484400587 ) ) ;
#12943=CARTESIAN_POINT ( 'NONE',  ( -9.485644917226064621, -49.78943610649189822, -17.51268299892230829 ) ) ;
#12946=ORIENTED_EDGE ( 'NONE', *, *, #3796, .T. ) ;
#12951=ORIENTED_EDGE ( 'NONE', *, *, #1787, .T. ) ;
#12969=CARTESIAN_POINT ( 'NONE',  ( 7.500300139189000070, -37.00737899243799944, 49.12071670408379731 ) ) ;
#12975=CARTESIAN_POINT ( 'NONE',  ( -15.49969986081099371, -23.50737899243800300, 56.85231026484400019 ) ) ;
#12984=CARTESIAN_POINT ( 'NONE',  ( -33.49969986081099904, -37.00737899243799944, -13.39525803434800011 ) ) ;
#12988=CARTESIAN_POINT ( 'NONE',  ( -5.499699860811003482, -46.50737899243799944, 47.50231026484399877 ) ) ;
#12995=DIRECTION ( 'NONE',  ( -1.054621095516909827E-16, -1.224646799147350002E-16, 1.000000000000000000 ) ) ;
#12997=ORIENTED_EDGE ( 'NONE', *, *, #9574, .F. ) ;
#13007=EDGE_CURVE ( 'NONE', #1679, #2810, #4016, .T. ) ;
#13012=EDGE_CURVE ( 'NONE', #2455, #12888, #5956, .T. ) ;
#13017=ORIENTED_EDGE ( 'NONE', *, *, #12630, .T. ) ;
#13018=CARTESIAN_POINT ( 'NONE',  ( -13.68042463183279089, -52.30222829753689950, -17.95442675827648316 ) ) ;
#13020=CARTESIAN_POINT ( 'NONE',  ( -35.22389609106763686, -38.22985747236961629, 51.39598352406615334 ) ) ;
#13031=CARTESIAN_POINT ( 'NONE',  ( 7.500300139189000070, -42.00737899243800655, 19.50231026484400587 ) ) ;
#13032=AXIS2_PLACEMENT_3D ( 'NONE', #7960, #5675, #1163 ) ;
#13040=CARTESIAN_POINT ( 'NONE',  ( 2.638979504099960405, -40.83713880673332142, -13.31900631518413824 ) ) ;
#13046=CARTESIAN_POINT ( 'NONE',  ( -7.499699860810999041, -19.50737899243799589, 54.00231026484400587 ) ) ;
#13047=CARTESIAN_POINT ( 'NONE',  ( -15.49969986081099727, -36.50737899243799944, 2.502310264843996546 ) ) ;
#13052=AXIS2_PLACEMENT_3D ( 'NONE', #10366, #12831, #4714 ) ;
#13054=DIRECTION ( 'NONE',  ( 1.000000000000000000, -1.291538348938060198E-32, 1.054621095516909827E-16 ) ) ;
#13055=VERTEX_POINT ( 'NONE', #3614 ) ;
#13061=CARTESIAN_POINT ( 'NONE',  ( -22.68580030561789940, -40.95256572998779632, 56.30791217491542966 ) ) ;
#13063=CARTESIAN_POINT ( 'NONE',  ( -10.02866676776782917, -38.66483879159430614, -17.59691272929029893 ) ) ;
#13066=CARTESIAN_POINT ( 'NONE',  ( -15.49969986081099904, -57.00737899243800655, 19.50231026484399877 ) ) ;
#13067=AXIS2_PLACEMENT_3D ( 'NONE', #7586, #8807, #632 ) ;
#13070=CARTESIAN_POINT ( 'NONE',  ( -15.49969986081099194, -27.00737899243800300, 19.50231026484399877 ) ) ;
#13075=DIRECTION ( 'NONE',  ( 0.000000000000000000, 1.700257036304450134E-17, -1.000000000000000000 ) ) ;
#13078=CARTESIAN_POINT ( 'NONE',  ( -7.510805671289423557, -44.08454136026598746, -6.142818529867362543 ) ) ;
#13082=PLANE ( 'NONE',  #9156 ) ;
#13090=CARTESIAN_POINT ( 'NONE',  ( -34.15367539102294359, -39.53260173292695612, 52.03355220560322181 ) ) ;
#13109=EDGE_CURVE ( 'NONE', #1528, #1516, #6550, .T. ) ;
#13143=DIRECTION ( 'NONE',  ( 0.000000000000000000, -1.000000000000000000, -1.224646799147350002E-16 ) ) ;
#13147=DIRECTION ( 'NONE',  ( 0.000000000000000000, -1.000000000000000000, -1.224646799147350002E-16 ) ) ;
#13156=VERTEX_POINT ( 'NONE', #3197 ) ;
#13158=ORIENTED_EDGE ( 'NONE', *, *, #1293, .F. ) ;
#13160=VECTOR ( 'NONE', #12830, 1000.000000000000000 ) ;
#13164=CARTESIAN_POINT ( 'NONE',  ( -7.836123178633778608, -47.48973556348496317, 17.20209991677158357 ) ) ;
#13169=CARTESIAN_POINT ( 'NONE',  ( -15.49969986081099904, -52.50737899243800655, -13.49768973515600656 ) ) ;
#13173=EDGE_LOOP ( 'NONE', ( #13502, #12019, #5371, #399 ) ) ;
#13174=CARTESIAN_POINT ( 'NONE',  ( -33.49969986081099904, -42.00737899243800655, -13.39525803434800011 ) ) ;
#13175=ORIENTED_EDGE ( 'NONE', *, *, #6730, .F. ) ;
#13181=DIRECTION ( 'NONE',  ( -1.734723475976805615E-16, 0.000000000000000000, 1.000000000000000000 ) ) ;
#13194=VERTEX_POINT ( 'NONE', #9002 ) ;
#13196=DIRECTION ( 'NONE',  ( 0.000000000000000000, 1.850371707708594316E-16, -1.000000000000000000 ) ) ;
#13205=DIRECTION ( 'NONE',  ( 1.000000000000000000, 0.000000000000000000, 0.000000000000000000 ) ) ;
#13209=ORIENTED_EDGE ( 'NONE', *, *, #1013, .T. ) ;
#13210=CARTESIAN_POINT ( 'NONE',  ( -23.49969986081099904, -44.50737899243799944, 19.50231026484399877 ) ) ;
#13212=CARTESIAN_POINT ( 'NONE',  ( -23.49969986081099904, -44.50737899243799944, -5.497689735156002122 ) ) ;
#13213=VERTEX_POINT ( 'NONE', #5712 ) ;
#13215=CARTESIAN_POINT ( 'NONE',  ( -23.49969986081100259, -44.50737899243799944, 56.13904046828872652 ) ) ;
#13216=EDGE_LOOP ( 'NONE', ( #7396, #6797 ) ) ;
#13238=CARTESIAN_POINT ( 'NONE',  ( -7.503901077028573674, -48.99487332462108213, 19.24414095425641946 ) ) ;
#13241=ORIENTED_EDGE ( 'NONE', *, *, #9892, .T. ) ;
#13242=CARTESIAN_POINT ( 'NONE',  ( -10.21329888696127419, -50.53437901354443085, -17.62507332399013293 ) ) ;
#13248=CARTESIAN_POINT ( 'NONE',  ( -33.58068771901564276, -41.10853556843252221, -13.35081987796131031 ) ) ;
#13252=CARTESIAN_POINT ( 'NONE',  ( -15.49969986081100259, -19.50737899243800300, 54.00231026484400587 ) ) ;
#13272=EDGE_CURVE ( 'NONE', #14077, #5522, #10266, .T. ) ;
#13282=FACE_OUTER_BOUND ( 'NONE', #7983, .T. ) ;
#13283=ORIENTED_EDGE ( 'NONE', *, *, #2707, .T. ) ;
#13286=ORIENTED_EDGE ( 'NONE', *, *, #2780, .F. ) ;
#13291=VECTOR ( 'NONE', #4752, 1000.000000000000000 ) ;
#13292=AXIS2_PLACEMENT_3D ( 'NONE', #11141, #1884, #11363 ) ;
#13297=CARTESIAN_POINT ( 'NONE',  ( -9.755182731580834599, -21.69540791116318346, 56.55967645960267021 ) ) ;
#13308=CARTESIAN_POINT ( 'NONE',  ( -11.90127153857799769, -52.50737899243803497, 11.50231026484396857 ) ) ;
#13311=COLOUR_RGB ( '', 0.66274510, 0.83137255, 0.94901961) ;
#13324=CYLINDRICAL_SURFACE ( 'NONE', #4485, 2.500000000000000000 ) ;
#13344=LINE ( 'NONE', #7588, #7547 ) ;
#13354=CARTESIAN_POINT ( 'NONE',  ( 2.500300139188996074, -46.50737899243799944, 47.50231026484399877 ) ) ;
#13359=EDGE_CURVE ( 'NONE', #10020, #3526, #5934, .T. ) ;
#13362=CARTESIAN_POINT ( 'NONE',  ( -11.00816613584963299, -22.44192803192691343, 56.73235138750358431 ) ) ;
#13363=DIRECTION ( 'NONE',  ( 0.000000000000000000, 0.000000000000000000, 1.000000000000000000 ) ) ;
#13366=DIRECTION ( 'NONE',  ( 0.000000000000000000, 0.000000000000000000, -1.000000000000000000 ) ) ;
#13377=CARTESIAN_POINT ( 'NONE',  ( -5.499699860811004370, -46.50737899243799944, 42.00231026484399166 ) ) ;
#13384=CARTESIAN_POINT ( 'NONE',  ( -7.607412389351752680, -48.63717025145547979, 18.15312534442707815 ) ) ;
#13393=CARTESIAN_POINT ( 'NONE',  ( -33.78790396967208665, -40.33206847766481928, -13.23593384171632259 ) ) ;
#13406=CARTESIAN_POINT ( 'NONE',  ( -7.499699860810997265, -44.50737899243797813, 46.00231026484399877 ) ) ;
#13408=DIRECTION ( 'NONE',  ( 0.000000000000000000, 1.000000000000000000, 1.224646799147350002E-16 ) ) ;
#13422=AXIS2_PLACEMENT_3D ( 'NONE', #13031, #7029, #10720 ) ;
#13423=EDGE_CURVE ( 'NONE', #5628, #5678, #8384, .T. ) ;
#13429=DIRECTION ( 'NONE',  ( 1.054621095516909827E-16, -1.224646799147350002E-16, 1.000000000000000000 ) ) ;
#13431=EDGE_LOOP ( 'NONE', ( #14315, #3445, #14778, #14005 ) ) ;
#13434=CARTESIAN_POINT ( 'NONE',  ( -17.58380395184910228, -52.23561682427189368, 56.94520027470884571 ) ) ;
#13437=VECTOR ( 'NONE', #1502, 1000.000000000000000 ) ;
#13441=EDGE_CURVE ( 'NONE', #13156, #12480, #8617, .T. ) ;
#13444=CARTESIAN_POINT ( 'NONE',  ( -15.49969986081099194, -36.50737899243799944, 11.50231026484399699 ) ) ;
#13458=VECTOR ( 'NONE', #11868, 1000.000000000000000 ) ;
#13466=CARTESIAN_POINT ( 'NONE',  ( -35.04849813642518086, -38.38910658708451251, -12.49920242367386791 ) ) ;
#13473=ADVANCED_FACE ( 'NONE', ( #3950 ), #9766, .F. ) ;
#13477=AXIS2_PLACEMENT_3D ( 'NONE', #5376, #11196, #1936 ) ;
#13500=FACE_OUTER_BOUND ( 'NONE', #7763, .T. ) ;
#13502=ORIENTED_EDGE ( 'NONE', *, *, #3796, .F. ) ;
#13523=DIRECTION ( 'NONE',  ( -1.000000000000000000, -3.700743415417187646E-16, 0.000000000000000000 ) ) ;
#13535=CARTESIAN_POINT ( 'NONE',  ( -7.661016837782100630, -46.08616143870106185, -3.031138187048190158 ) ) ;
#13537=ORIENTED_EDGE ( 'NONE', *, *, #10648, .F. ) ;
#13540=ORIENTED_EDGE ( 'NONE', *, *, #10868, .T. ) ;
#13544=CARTESIAN_POINT ( 'NONE',  ( -7.499699860810998153, -44.50737899243799944, 56.13904046828873362 ) ) ;
#13545=EDGE_CURVE ( 'NONE', #9803, #14198, #3098, .T. ) ;
#13554=CARTESIAN_POINT ( 'NONE',  ( -7.512109644807973829, -44.06143319563968674, 43.96819400509183140 ) ) ;
#13558=DIRECTION ( 'NONE',  ( 0.000000000000000000, 0.000000000000000000, 1.000000000000000000 ) ) ;
#13559=EDGE_LOOP ( 'NONE', ( #10306, #11738 ) ) ;
#13560=ORIENTED_EDGE ( 'NONE', *, *, #7943, .F. ) ;
#13568=ADVANCED_FACE ( 'NONE', ( #10051 ), #11065, .F. ) ;
#13575=LINE ( 'NONE', #10112, #6527 ) ;
#13576=ORIENTED_EDGE ( 'NONE', *, *, #10197, .T. ) ;
#13581=ADVANCED_FACE ( 'NONE', ( #658, #2875 ), #6679, .T. ) ;
#13583=CARTESIAN_POINT ( 'NONE',  ( -15.23828507852217129, -36.50737899243799944, 57.00231026484397745 ) ) ;
#13585=CARTESIAN_POINT ( 'NONE',  ( -7.499699860810999041, -44.50737899243799944, -17.13441993860073964 ) ) ;
#13588=ADVANCED_FACE ( 'NONE', ( #14804 ), #886, .F. ) ;
#13597=CARTESIAN_POINT ( 'NONE',  ( 2.500300139188999182, -51.00737899243799944, 52.39987856403599409 ) ) ;
#13599=CARTESIAN_POINT ( 'NONE',  ( -7.499699860810999041, -19.50737899243799589, 48.00231026484399877 ) ) ;
#13610=CARTESIAN_POINT ( 'NONE',  ( -7.510639545435999764, -44.94673998318546637, -3.544435685291067895 ) ) ;
#13619=CIRCLE ( 'NONE', #6510, 2.999999999999999112 ) ;
#13620=CYLINDRICAL_SURFACE ( 'NONE', #3588, 3.000000000000002665 ) ;
#13646=DIRECTION ( 'NONE',  ( 0.000000000000000000, -1.000000000000000000, -1.224646799147350002E-16 ) ) ;
#13652=DIRECTION ( 'NONE',  ( 1.445602896647339656E-16, 0.000000000000000000, -1.000000000000000000 ) ) ;
#13655=CARTESIAN_POINT ( 'NONE',  ( -10.61847719068383178, -38.14777797243608859, 56.68582056335808517 ) ) ;
#13657=FACE_BOUND ( 'NONE', #13785, .T. ) ;
#13666=CARTESIAN_POINT ( 'NONE',  ( -5.499699860811000818, -46.50737899243799944, 19.50231026484399877 ) ) ;
#13673=CARTESIAN_POINT ( 'NONE',  ( -22.67768377378909506, -40.96543783778685821, -17.30451537288594110 ) ) ;
#13677=CIRCLE ( 'NONE', #6080, 2.500000000000002220 ) ;
#13679=CARTESIAN_POINT ( 'NONE',  ( -7.638565634192136855, -48.52246210452846498, 20.98308540249201926 ) ) ;
#13685=CARTESIAN_POINT ( 'NONE',  ( -7.508516329967514835, -44.90912954173229821, -3.575286200065592279 ) ) ;
#13696=CARTESIAN_POINT ( 'NONE',  ( -7.796313671854394833, -46.67229257320486369, 42.00231026484398456 ) ) ;
#13697=DIRECTION ( 'NONE',  ( -3.632077277826439854E-16, 1.000000000000000000, 0.000000000000000000 ) ) ;
#13701=ORIENTED_EDGE ( 'NONE', *, *, #4125, .T. ) ;
#13707=ORIENTED_EDGE ( 'NONE', *, *, #6061, .F. ) ;
#13708=CARTESIAN_POINT ( 'NONE',  ( -15.49969986081099194, -32.00737899243799944, 19.50231026484399166 ) ) ;
#13715=FACE_OUTER_BOUND ( 'NONE', #6815, .T. ) ;
#13716=FACE_OUTER_BOUND ( 'NONE', #14698, .T. ) ;
#13722=VERTEX_POINT ( 'NONE', #1182 ) ;
#13726=CARTESIAN_POINT ( 'NONE',  ( -8.211338606302485132, -41.19849018162404519, 56.28736606044791557 ) ) ;
#13738=CARTESIAN_POINT ( 'NONE',  ( -15.49969986081099904, -27.00737899243800300, -5.497689735156002122 ) ) ;
#13743=CARTESIAN_POINT ( 'NONE',  ( -22.29394651601237953, -40.27574555278066981, -17.37736014901681969 ) ) ;
#13746=ORIENTED_EDGE ( 'NONE', *, *, #10282, .T. ) ;
#13747=FACE_OUTER_BOUND ( 'NONE', #4945, .T. ) ;
#13750=EDGE_CURVE ( 'NONE', #9567, #234, #12802, .T. ) ;
#13752=CARTESIAN_POINT ( 'NONE',  ( -5.499699860811004370, -46.50737899243799944, 44.50231026484399877 ) ) ;
#13758=CARTESIAN_POINT ( 'NONE',  ( -7.509222570460704738, -44.92217572422880778, -3.564520568178003668 ) ) ;
#13760=ORIENTED_EDGE ( 'NONE', *, *, #10648, .T. ) ;
#13764=CARTESIAN_POINT ( 'NONE',  ( -8.567699421354552314, -48.50933269009345139, 56.35625304898181298 ) ) ;
#13772=CARTESIAN_POINT ( 'NONE',  ( -8.826344180179512833, -48.91964147717249034, 43.82441874199299292 ) ) ;
#13773=DIRECTION ( 'NONE',  ( 0.000000000000000000, 1.000000000000000000, 1.224646799147350002E-16 ) ) ;
#13782=ORIENTED_EDGE ( 'NONE', *, *, #7342, .T. ) ;
#13783=CARTESIAN_POINT ( 'NONE',  ( -15.49969986081099371, -26.50737899243800300, 56.85231026484400019 ) ) ;
#13785=EDGE_LOOP ( 'NONE', ( #1124, #4301, #1007, #9641 ) ) ;
#13789=VECTOR ( 'NONE', #2130, 1000.000000000000000 ) ;
#13795=CARTESIAN_POINT ( 'NONE',  ( -23.39591611362797963, -45.81830490939771039, -17.15696593335874454 ) ) ;
#13803=ORIENTED_EDGE ( 'NONE', *, *, #14486, .T. ) ;
#13804=CARTESIAN_POINT ( 'NONE',  ( -8.706569105308981094, -40.27405685900905752, 56.38218252410854348 ) ) ;
#13810=EDGE_CURVE ( 'NONE', #6515, #11225, #4364, .T. ) ;
#13814=CARTESIAN_POINT ( 'NONE',  ( -15.49969986081099727, -52.50737899243799944, 2.502310264843994769 ) ) ;
#13817=ORIENTED_EDGE ( 'NONE', *, *, #14251, .T. ) ;
#13820=DIRECTION ( 'NONE',  ( 0.000000000000000000, -1.000000000000000000, -1.224646799147350002E-16 ) ) ;
#13845=VECTOR ( 'NONE', #5454, 1000.000000000000000 ) ;
#13853=AXIS2_PLACEMENT_3D ( 'NONE', #8171, #8400, #8248 ) ;
#13857=ORIENTED_EDGE ( 'NONE', *, *, #9594, .F. ) ;
#13861=ADVANCED_FACE ( 'NONE', ( #4208 ), #14836, .F. ) ;
#13867=CARTESIAN_POINT ( 'NONE',  ( -15.49969986081099371, -52.50737899243799944, -17.99768973515599768 ) ) ;
#13900=ADVANCED_FACE ( 'NONE', ( #9936 ), #14612, .T. ) ;
#13903=AXIS2_PLACEMENT_3D ( 'NONE', #7077, #2662, #13075 ) ;
#13911=AXIS2_PLACEMENT_3D ( 'NONE', #3910, #5274, #10875 ) ;
#13947=VERTEX_POINT ( 'NONE', #10395 ) ;
#13953=CARTESIAN_POINT ( 'NONE',  ( -15.49969986081099016, -27.00737899243800300, 27.50231026484399877 ) ) ;
#13955=VECTOR ( 'NONE', #2553, 1000.000000000000000 ) ;
#13959=ORIENTED_EDGE ( 'NONE', *, *, #11309, .T. ) ;
#13961=CARTESIAN_POINT ( 'NONE',  ( -5.499699860811003482, -46.50737899243799944, 41.50231026484399166 ) ) ;
#13964=DIRECTION ( 'NONE',  ( 0.000000000000000000, 0.000000000000000000, 1.000000000000000000 ) ) ;
#13965=ADVANCED_FACE ( 'NONE', ( #8085 ), #11470, .F. ) ;
#13976=DIRECTION ( 'NONE',  ( 1.054621095516909827E-16, -1.224646799147350002E-16, 1.000000000000000000 ) ) ;
#13978=AXIS2_PLACEMENT_3D ( 'NONE', #279, #11898, #10602 ) ;
#13982=( BOUNDED_CURVE ( )  B_SPLINE_CURVE ( 3, ( #7806, #12493, #6663, #11346 ),
 .UNSPECIFIED., .F., .F. ) 
 B_SPLINE_CURVE_WITH_KNOTS ( ( 4, 4 ),
 ( 5.060245233341797544, 5.259239931080632147 ),
 .UNSPECIFIED. ) 
 CURVE ( )  GEOMETRIC_REPRESENTATION_ITEM ( )  RATIONAL_B_SPLINE_CURVE ( ( 1.000000000000000000, 0.9967028139718016044, 0.9967028139718016044, 1.000000000000000000 ) ) 
 REPRESENTATION_ITEM ( '' )  );
#13986=EDGE_CURVE ( 'NONE', #9646, #8988, #11618, .T. ) ;
#14005=ORIENTED_EDGE ( 'NONE', *, *, #13986, .F. ) ;
#14020=CARTESIAN_POINT ( 'NONE',  ( -23.24172680504385369, -46.58969747883803336, -17.18995143628628952 ) ) ;
#14023=CARTESIAN_POINT ( 'NONE',  ( 3.154275669408413307, -39.53260173292035518, -13.02893167591090773 ) ) ;
#14038=CARTESIAN_POINT ( 'NONE',  ( -7.694327897266501459, -46.24447382526680173, 21.98901576030363358 ) ) ;
#14046=ORIENTED_EDGE ( 'NONE', *, *, #7928, .T. ) ;
#14051=ORIENTED_EDGE ( 'NONE', *, *, #283, .T. ) ;
#14056=CARTESIAN_POINT ( 'NONE',  ( -23.49969986081099904, -44.50737899243799944, -5.497689735156002122 ) ) ;
#14059=FACE_OUTER_BOUND ( 'NONE', #3202, .T. ) ;
#14064=ORIENTED_EDGE ( 'NONE', *, *, #4819, .F. ) ;
#14071=( BOUNDED_CURVE ( )  B_SPLINE_CURVE ( 3, ( #13444, #733, #9840, #11064 ),
 .UNSPECIFIED., .F., .F. ) 
 B_SPLINE_CURVE_WITH_KNOTS ( ( 4, 4 ),
 ( 3.141592653589792672, 4.712388980384689674 ),
 .UNSPECIFIED. ) 
 CURVE ( )  GEOMETRIC_REPRESENTATION_ITEM ( )  RATIONAL_B_SPLINE_CURVE ( ( 1.000000000000000000, 0.8047378541243649375, 0.8047378541243649375, 1.000000000000000000 ) ) 
 REPRESENTATION_ITEM ( '' )  );
#14074=CARTESIAN_POINT ( 'NONE',  ( -7.844836682715700782, -47.42038978965683782, -7.826127288787263936 ) ) ;
#14075=CARTESIAN_POINT ( 'NONE',  ( -7.886584594865190034, -46.96511696614950182, -7.955427708867500058 ) ) ;
#14077=VERTEX_POINT ( 'NONE', #1520 ) ;
#14089=DIRECTION ( 'NONE',  ( 0.000000000000000000, 1.850371707708594316E-16, -1.000000000000000000 ) ) ;
#14094=B_SPLINE_CURVE_WITH_KNOTS ( 'NONE', 3,
 ( #1028, #10354, #15023, #3399, #6897, #11579, #10429, #15096, #4621, #12819, #2330, #804, #3549, #2406, #10659, #3779, #2555, #37 ),
 .UNSPECIFIED., .F., .F.,
 ( 4, 2, 2, 2, 1, 1, 2, 2, 2, 4 ),
 ( 0.000000000000000000, 0.2500000000000217604, 0.3750000000000327516, 0.4375000000000378031, 0.4687500000000399125, 0.4843750000000400791, 0.4921875000000398015, 0.5000000000000394129, 0.7500000000000197620, 1.000000000000000000 ),
 .UNSPECIFIED. ) ;
#14102=CARTESIAN_POINT ( 'NONE',  ( 5.055282432709286233, -37.64246294776327062, 50.86739471227122067 ) ) ;
#14111=CARTESIAN_POINT ( 'NONE',  ( -7.654737080345056732, -48.45581950336406862, -3.931260860926701461 ) ) ;
#14115=AXIS2_PLACEMENT_3D ( 'NONE', #13666, #815, #3331 ) ;
#14122=CARTESIAN_POINT ( 'NONE',  ( -33.49969986081099904, -42.00737899243800655, -13.39525803434800011 ) ) ;
#14130=CIRCLE ( 'NONE', #455, 2.499999999999998668 ) ;
#14131=CARTESIAN_POINT ( 'NONE',  ( -7.494898247900367849, -44.62174188576448586, 17.84928634147309268 ) ) ;
#14135=LINE ( 'NONE', #10533, #3599 ) ;
#14154=CYLINDRICAL_SURFACE ( 'NONE', #14352, 8.000000000000000000 ) ;
#14155=CARTESIAN_POINT ( 'NONE',  ( -35.19389501775997786, -38.25609885807658372, 51.41451777256275335 ) ) ;
#14173=AXIS2_PLACEMENT_3D ( 'NONE', #2181, #2027, #11506 ) ;
#14175=CARTESIAN_POINT ( 'NONE',  ( 5.196266986419307621, -37.55864118711512845, -11.77116662607953046 ) ) ;
#14188=CARTESIAN_POINT ( 'NONE',  ( -7.501950027729723303, -44.50597529135383468, 20.99749114769749880 ) ) ;
#14190=ORIENTED_EDGE ( 'NONE', *, *, #10982, .T. ) ;
#14194=ORIENTED_EDGE ( 'NONE', *, *, #13750, .F. ) ;
#14198=VERTEX_POINT ( 'NONE', #9702 ) ;
#14208=CARTESIAN_POINT ( 'NONE',  ( -0.3742611254310204694, -27.95036676736704706, 53.90694524323487258 ) ) ;
#14220=CARTESIAN_POINT ( 'NONE',  ( -11.49119621977820671, -37.57910197549196596, 56.78818114396622718 ) ) ;
#14221=FACE_OUTER_BOUND ( 'NONE', #5198, .T. ) ;
#14228=VECTOR ( 'NONE', #10474, 1000.000000000000000 ) ;
#14231=CARTESIAN_POINT ( 'NONE',  ( -11.95839784354461521, -51.68564174154704460, -17.83082277104466939 ) ) ;
#14232=CARTESIAN_POINT ( 'NONE',  ( -33.73358454970886555, -40.49459960334031905, 52.27083934352044992 ) ) ;
#14251=EDGE_CURVE ( 'NONE', #3246, #10391, #5596, .T. ) ;
#14259=ORIENTED_EDGE ( 'NONE', *, *, #4232, .F. ) ;
#14268=CARTESIAN_POINT ( 'NONE',  ( -7.662963790453773072, -48.42200951437354206, -7.105263616372978319 ) ) ;
#14278=( LENGTH_UNIT ( ) NAMED_UNIT ( * ) SI_UNIT ( .MILLI., .METRE. ) );
#14288=CARTESIAN_POINT ( 'NONE',  ( 2.500300139188999626, -46.50737899243799944, 16.50231026484399877 ) ) ;
#14291=CARTESIAN_POINT ( 'NONE',  ( -15.49969986081099016, -27.00737899243800300, 27.50231026484399877 ) ) ;
#14292=CARTESIAN_POINT ( 'NONE',  ( -7.754954776104139746, -46.50766419030464505, -2.997807438439666239 ) ) ;
#14306=CARTESIAN_POINT ( 'NONE',  ( -9.152138177982815037, -49.38359113951253221, -17.45695168481910287 ) ) ;
#14311=EDGE_LOOP ( 'NONE', ( #6644, #11386 ) ) ;
#14315=ORIENTED_EDGE ( 'NONE', *, *, #2459, .F. ) ;
#14335=ORIENTED_EDGE ( 'NONE', *, *, #960, .T. ) ;
#14338=PLANE ( 'NONE',  #3188 ) ;
#14344=CARTESIAN_POINT ( 'NONE',  ( -7.869402401354462562, -47.25089185753165566, -3.093175506660042817 ) ) ;
#14351=DIRECTION ( 'NONE',  ( 1.000000000000000000, -1.291538348938060198E-32, 1.054621095516909827E-16 ) ) ;
#14352=AXIS2_PLACEMENT_3D ( 'NONE', #1297, #463, #7328 ) ;
#14358=LINE ( 'NONE', #12988, #3411 ) ;
#14359=CARTESIAN_POINT ( 'NONE',  ( -10.98945933209236969, -22.43249828447867245, 56.73009184860239884 ) ) ;
#14361=CARTESIAN_POINT ( 'NONE',  ( -7.512172356294475328, -44.98005919120003426, 17.52071913701680828 ) ) ;
#14367=ORIENTED_EDGE ( 'NONE', *, *, #3691, .T. ) ;
#14372=CARTESIAN_POINT ( 'NONE',  ( -7.754930580632606762, -46.50765881518451295, 22.00225574842814424 ) ) ;
#14378=CARTESIAN_POINT ( 'NONE',  ( -7.773685182324180154, -47.89679818372218278, 17.41897699471824623 ) ) ;
#14382=CARTESIAN_POINT ( 'NONE',  ( -7.551915124174499283, -45.55891546459999830, -17.14593156766008164 ) ) ;
#14392=DIRECTION ( 'NONE',  ( 1.445602896647339656E-16, 0.000000000000000000, -1.000000000000000000 ) ) ;
#14406=EDGE_CURVE ( 'NONE', #1735, #10639, #13677, .T. ) ;
#14418=DIRECTION ( 'NONE',  ( -0.000000000000000000, 1.000000000000000000, 0.000000000000000000 ) ) ;
#14435=ORIENTED_EDGE ( 'NONE', *, *, #3341, .F. ) ;
#14436=B_SPLINE_CURVE_WITH_KNOTS ( 'NONE', 3,
 ( #7493, #11017, #7421, #2836 ),
 .UNSPECIFIED., .F., .F.,
 ( 4, 4 ),
 ( 0.000000000000000000, 0.1213360741398818166 ),
 .UNSPECIFIED. ) ;
#14448=DIRECTION ( 'NONE',  ( 1.000000000000000000, 0.000000000000000000, 0.000000000000000000 ) ) ;
#14450=CARTESIAN_POINT ( 'NONE',  ( -12.92091935695870042, -52.08489029401035708, -17.90976127491029146 ) ) ;
#14452=CARTESIAN_POINT ( 'NONE',  ( -34.37762275815202173, -39.17044586891318403, 51.90428018001587418 ) ) ;
#14455=VERTEX_POINT ( 'NONE', #4495 ) ;
#14456=CARTESIAN_POINT ( 'NONE',  ( -35.14379750997561302, -38.30087877078398151, -12.44075990407947607 ) ) ;
#14467=CARTESIAN_POINT ( 'NONE',  ( -33.49969986081099904, -37.00737899243799944, 19.50231026484398811 ) ) ;
#14471=DIRECTION ( 'NONE',  ( -1.054621095516909827E-16, 1.224646799147350002E-16, -1.000000000000000000 ) ) ;
#14476=EDGE_LOOP ( 'NONE', ( #13017, #12951 ) ) ;
#14486=EDGE_CURVE ( 'NONE', #14455, #9903, #6567, .T. ) ;
#14488=CARTESIAN_POINT ( 'NONE',  ( -15.49969986081099727, -27.00737899243800300, 2.502310264843997878 ) ) ;
#14492=CARTESIAN_POINT ( 'NONE',  ( -15.49969986081099904, -57.00737899243800655, 19.50231026484399877 ) ) ;
#14497=CARTESIAN_POINT ( 'NONE',  ( -20.79164517123715683, -50.52944030466328940, 56.62889509689365042 ) ) ;
#14519=LINE ( 'NONE', #9851, #11077 ) ;
#14521=ORIENTED_EDGE ( 'NONE', *, *, #11827, .T. ) ;
#14524=CARTESIAN_POINT ( 'NONE',  ( -7.707857435417036385, -48.23250629231411324, 17.69147438052686994 ) ) ;
#14528=ORIENTED_EDGE ( 'NONE', *, *, #5445, .T. ) ;
#14534=CARTESIAN_POINT ( 'NONE',  ( -34.94125367352354061, -38.49305635555177929, -12.56456997079345506 ) ) ;
#14538=DIRECTION ( 'NONE',  ( 1.000000000000000000, -1.291538348938060198E-32, 1.054621095516909827E-16 ) ) ;
#14539=EDGE_CURVE ( 'NONE', #2347, #11156, #3653, .T. ) ;
#14540=ADVANCED_FACE ( 'NONE', ( #8227 ), #7380, .T. ) ;
#14545=CARTESIAN_POINT ( 'NONE',  ( -7.512805849530849400, -44.04964101872670312, 19.04457229113268113 ) ) ;
#14547=PLANE ( 'NONE',  #4723 ) ;
#14552=CARTESIAN_POINT ( 'NONE',  ( -7.517675258046085496, -45.05616182903360567, -7.535809151347679702 ) ) ;
#14553=ORIENTED_EDGE ( 'NONE', *, *, #393, .T. ) ;
#14565=CARTESIAN_POINT ( 'NONE',  ( -38.49969986081099904, -42.00737899243800655, 19.50231026484398811 ) ) ;
#14578=CARTESIAN_POINT ( 'NONE',  ( -10.70529993155776083, -22.28872569541405113, 56.69565590118975962 ) ) ;
#14579=EDGE_CURVE ( 'NONE', #2810, #12214, #7223, .T. ) ;
#14583=FACE_OUTER_BOUND ( 'NONE', #5455, .T. ) ;
#14584=CIRCLE ( 'NONE', #4321, 37.50000000000000711 ) ;
#14591=CARTESIAN_POINT ( 'NONE',  ( -7.795056982475612628, -46.66304653480354858, 22.00230981020063581 ) ) ;
#14605=CARTESIAN_POINT ( 'NONE',  ( -33.65607387164132547, -40.75537920815241932, -13.30924300046305397 ) ) ;
#14607=B_SPLINE_CURVE_WITH_KNOTS ( 'NONE', 3,
 ( #6670, #10195, #11577, #3089, #802, #9047, #2099, #6741, #954, #5607, #3620, #187, #9433, #8125, #10734, #10507, #11725, #11962, #2328, #12817, #4699, #6963, #8278, #10581, #116, #14102, #9585, #261, #5902, #2474, #8357, #12887, #11651, #1480, #12969 ),
 .UNSPECIFIED., .F., .F.,
 ( 4, 2, 2, 2, 2, 2, 2, 2, 2, 1, 1, 2, 2, 2, 1, 1, 1, 2, 2, 4 ),
 ( 0.000000000000000000, 0.06250000000000119349, 0.09375000000000185962, 0.1250000000000025258, 0.1875000000000059119, 0.2187500000000087153, 0.2500000000000114908, 0.3750000000000204836, 0.4375000000000254796, 0.4687500000000274780, 0.4843750000000288103, 0.4921875000000295319, 0.5000000000000303091, 0.6250000000000239808, 0.6875000000000202061, 0.7187500000000189848, 0.7343750000000175415, 0.7421875000000172085, 0.7500000000000167644, 1.000000000000000000 ),
 .UNSPECIFIED. ) ;
#14612=CYLINDRICAL_SURFACE ( 'NONE', #12776, 37.49999999999999289 ) ;
#14619=CARTESIAN_POINT ( 'NONE',  ( -7.506371897368028456, -44.17798263326779562, 43.58480693617389079 ) ) ;
#14620=ORIENTED_EDGE ( 'NONE', *, *, #12574, .T. ) ;
#14622=ORIENTED_EDGE ( 'NONE', *, *, #3311, .F. ) ;
#14624=CARTESIAN_POINT ( 'NONE',  ( -7.593870215980957461, -45.75074864731840307, -7.912782458232928917 ) ) ;
#14627=( GEOMETRIC_REPRESENTATION_CONTEXT ( 3 ) GLOBAL_UNCERTAINTY_ASSIGNED_CONTEXT ( ( #11702 ) ) GLOBAL_UNIT_ASSIGNED_CONTEXT ( ( #10339, #9113, #9184 ) ) REPRESENTATION_CONTEXT ( 'NONE', 'WORKASPACE' ) );
#14630=ORIENTED_EDGE ( 'NONE', *, *, #5882, .F. ) ;
#14635=B_SPLINE_CURVE_WITH_KNOTS ( 'NONE', 3,
 ( #9295, #2117, #8145, #6760, #4794, #7062, #7218, #5921, #13061, #12835, #7142, #9603, #5846, #2570, #1263, #363, #8295, #10755, #2646, #9378, #8220, #4944, #4872 ),
 .UNSPECIFIED., .F., .F.,
 ( 4, 2, 1, 2, 2, 2, 2, 2, 2, 2, 2, 4 ),
 ( 0.01260726791730938309, 0.01339567446202048762, 0.01418408100673159040, 0.01497248755144269493, 0.01576089409615379772, 0.01733770718557600329, 0.01891452027499820887, 0.02049133336442041098, 0.02127973990913151550, 0.02206814645384262003, 0.02364495954326482213, 0.02522177263268702771 ),
 .UNSPECIFIED. ) ;
#14642=EDGE_CURVE ( 'NONE', #11647, #10391, #14358, .T. ) ;
#14646=CARTESIAN_POINT ( 'NONE',  ( -7.497874475122997318, -44.50608669435617770, -6.993290823733421036 ) ) ;
#14648=CIRCLE ( 'NONE', #9995, 2.500000000000002220 ) ;
#14653=( BOUNDED_CURVE ( )  B_SPLINE_CURVE ( 3, ( #11234, #4045, #7624, #8851 ),
 .UNSPECIFIED., .F., .T. ) 
 B_SPLINE_CURVE_WITH_KNOTS ( ( 4, 4 ),
 ( 3.141592653589793116, 4.400121501412645131 ),
 .UNSPECIFIED. ) 
 CURVE ( )  GEOMETRIC_REPRESENTATION_ITEM ( )  RATIONAL_B_SPLINE_CURVE ( ( 1.000000000000000000, 0.8723071003127529366, 0.8723071003127529366, 1.000000000000000000 ) ) 
 REPRESENTATION_ITEM ( '' )  );
#14659=CARTESIAN_POINT ( 'NONE',  ( -15.42469986081099442, -23.50737899243800300, 56.85231026484400019 ) ) ;
#14671=CARTESIAN_POINT ( 'NONE',  ( -7.499699427612009472, -49.00737706678066274, 19.48780283923079537 ) ) ;
#14679=DIRECTION ( 'NONE',  ( 1.000000000000000000, -1.291538348938060198E-32, 1.054621095516909827E-16 ) ) ;
#14682=DIRECTION ( 'NONE',  ( -1.000000000000000000, 1.291538348938060198E-32, -1.054621095516909827E-16 ) ) ;
#14684=CARTESIAN_POINT ( 'NONE',  ( -15.49969986081099727, -36.50737899243799944, 2.502310264843996546 ) ) ;
#14688=CARTESIAN_POINT ( 'NONE',  ( -8.792249626181712685, -48.86814062846791984, 43.66295784926125378 ) ) ;
#14690=CARTESIAN_POINT ( 'NONE',  ( -15.49969986081099904, -44.50737899243799944, -109.5506571639849938 ) ) ;
#14698=EDGE_LOOP ( 'NONE', ( #8306, #4014, #1438, #12016, #11752, #5309 ) ) ;
#14699=ORIENTED_EDGE ( 'NONE', *, *, #12266, .T. ) ;
#14718=VERTEX_POINT ( 'NONE', #13585 ) ;
#14724=DIRECTION ( 'NONE',  ( 0.000000000000000000, 0.000000000000000000, 1.000000000000000000 ) ) ;
#14729=DIRECTION ( 'NONE',  ( 1.000000000000000000, -1.291538348938060198E-32, 1.054621095516909827E-16 ) ) ;
#14750=CARTESIAN_POINT ( 'NONE',  ( -7.705418609685459330, -48.24386234041415378, 21.32367631506333439 ) ) ;
#14767=PLANE ( 'NONE',  #5247 ) ;
#14772=DIRECTION ( 'NONE',  ( 1.000000000000000000, 0.000000000000000000, 0.000000000000000000 ) ) ;
#14776=ORIENTED_EDGE ( 'NONE', *, *, #2804, .F. ) ;
#14778=ORIENTED_EDGE ( 'NONE', *, *, #5588, .T. ) ;
#14782=DIRECTION ( 'NONE',  ( 0.000000000000000000, 0.000000000000000000, 1.000000000000000000 ) ) ;
#14783=EDGE_CURVE ( 'NONE', #11671, #855, #253, .T. ) ;
#14791=ORIENTED_EDGE ( 'NONE', *, *, #2614, .T. ) ;
#14804=FACE_OUTER_BOUND ( 'NONE', #1464, .T. ) ;
#14807=CARTESIAN_POINT ( 'NONE',  ( -7.886584594865180264, -46.96511696614940234, -3.039951761444701361 ) ) ;
#14815=AXIS2_PLACEMENT_3D ( 'NONE', #14690, #8870, #3057 ) ;
#14817=CARTESIAN_POINT ( 'NONE',  ( 4.000300139189000959, -20.37340439622240851, 51.53354502093799994 ) ) ;
#14820=CARTESIAN_POINT ( 'NONE',  ( -7.649802761028805520, -48.47628348355012662, 21.04316911978840210 ) ) ;
#14836=PLANE ( 'NONE',  #5182 ) ;
#14837=DIRECTION ( 'NONE',  ( 0.000000000000000000, 0.000000000000000000, 1.000000000000000000 ) ) ;
#14863=CARTESIAN_POINT ( 'NONE',  ( -19.50984199700181776, -51.43466821614173057, -17.78337838361071732 ) ) ;
#14876=CARTESIAN_POINT ( 'NONE',  ( -8.572300031023576850, -40.49742984648624855, 56.35711988542138329 ) ) ;
#14881=DIRECTION ( 'NONE',  ( -1.000000000000000000, 1.291538348938060198E-32, -1.054621095516909827E-16 ) ) ;
#14885=CARTESIAN_POINT ( 'NONE',  ( -8.992083836518995454, -50.38952316532486009, 0.3844544377308600214 ) ) ;
#14890=VERTEX_POINT ( 'NONE', #3173 ) ;
#14892=CARTESIAN_POINT ( 'NONE',  ( -17.06800750706793224, -36.64961894308596868, -17.96750743336168910 ) ) ;
#14915=CARTESIAN_POINT ( 'NONE',  ( -8.659108278886616716, -48.65678357935241394, 43.21545986666426842 ) ) ;
#14920=CARTESIAN_POINT ( 'NONE',  ( -31.89126067837590028, -25.75737899243799944, -17.99768973515599768 ) ) ;
#14935=CARTESIAN_POINT ( 'NONE',  ( -16.55482201156862487, -52.45476196004928227, -17.98636559174942562 ) ) ;
#14937=DIRECTION ( 'NONE',  ( 0.000000000000000000, 0.000000000000000000, 1.000000000000000000 ) ) ;
#14945=CARTESIAN_POINT ( 'NONE',  ( -8.995873580312741424, -39.84177233736869539, 56.43429974597158605 ) ) ;
#14947=CARTESIAN_POINT ( 'NONE',  ( -15.49969986081100259, -19.50737899243800300, -17.99768973515599768 ) ) ;
#14955=FACE_OUTER_BOUND ( 'NONE', #4133, .T. ) ;
#14958=ORIENTED_EDGE ( 'NONE', *, *, #8696, .F. ) ;
#14964=CARTESIAN_POINT ( 'NONE',  ( -23.08905235891587182, -41.92403831085029964, -17.22224902766740584 ) ) ;
#14967=CARTESIAN_POINT ( 'NONE',  ( -15.42469986081099442, -26.50737899243800300, 56.85231026484400019 ) ) ;
#14969=VECTOR ( 'NONE', #2397, 1000.000000000000000 ) ;
#14981=EDGE_LOOP ( 'NONE', ( #172, #6895, #12516, #9868 ) ) ;
#14993=CARTESIAN_POINT ( 'NONE',  ( -35.18004919290292776, -38.26834254388187162, 51.42305902976909948 ) ) ;
#14999=ORIENTED_EDGE ( 'NONE', *, *, #9140, .F. ) ;
#15003=DIRECTION ( 'NONE',  ( 0.000000000000000000, -1.000000000000000000, -1.224646799147350002E-16 ) ) ;
#15010=CARTESIAN_POINT ( 'NONE',  ( -22.42809723928562349, -48.51567270060554193, -17.35231326048090850 ) ) ;
#15023=CARTESIAN_POINT ( 'NONE',  ( -22.51561314124201374, -20.67385552401155380, 56.34133000697264748 ) ) ;
#15027=CARTESIAN_POINT ( 'NONE',  ( -7.527662185239785586, -45.17397162665944421, 21.61993551438897754 ) ) ;
#15036=EDGE_CURVE ( 'NONE', #5221, #3880, #2934, .T. ) ;
#15037=CARTESIAN_POINT ( 'NONE',  ( -23.44892144575882043, -43.46354585320516151, -17.14562330798139200 ) ) ;
#15075=ORIENTED_EDGE ( 'NONE', *, *, #4592, .T. ) ;
#15086=CARTESIAN_POINT ( 'NONE',  ( -20.16554002329735340, -51.01103853986323600, -17.70692683075240126 ) ) ;
#15096=CARTESIAN_POINT ( 'NONE',  ( -20.44297195033120929, -22.20066666004292699, 56.67562539687022394 ) ) ;
#15099=FACE_OUTER_BOUND ( 'NONE', #3223, .T. ) ;
#15102=CARTESIAN_POINT ( 'NONE',  ( -7.705950972875354132, -46.29720360269725177, 21.99401816995757386 ) ) ;
#15106=CARTESIAN_POINT ( 'NONE',  ( -7.502323095902962535, -44.76088757143082830, 42.70304391562847002 ) ) ;
ENDSEC;
END-ISO-10303-21;
